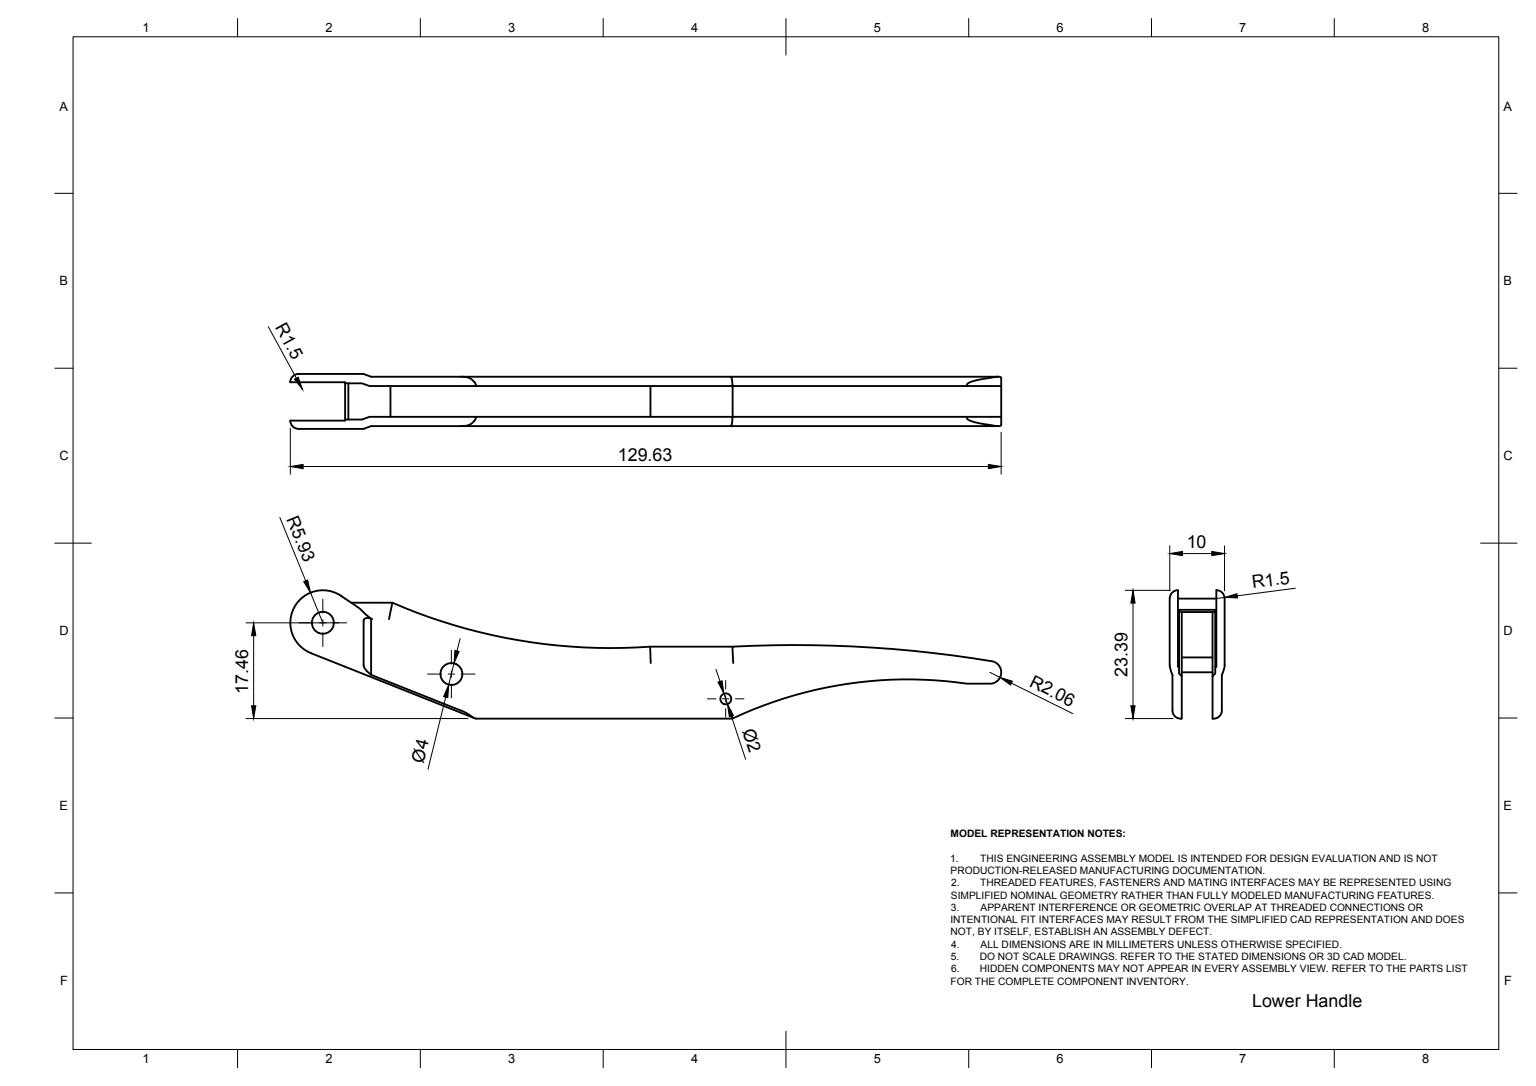
ISO-10303-21;
HEADER;
/* Generated by software containing ST-Developer
 * from STEP Tools, Inc. (www.steptools.com) 
 */

FILE_DESCRIPTION(
/* description */ ('STEP AP214'),
/* implementation_level */ '2;1');

FILE_NAME(
/* name */ 'Lower Handle.step',
/* time_stamp */ '2026-10-06T11:11:25-07:00',
/* author */ (''),
/* organization */ (''),
/* preprocessor_version */ 'ST-DEVELOPER v20.2',
/* originating_system */ 'Autodesk Translation Framework v15.15.0.0',
/* authorisation */ '');

FILE_SCHEMA (('AUTOMOTIVE_DESIGN { 1 0 10303 214 3 1 1 }'));
ENDSEC;

DATA;
#10=MECHANICAL_DESIGN_GEOMETRIC_PRESENTATION_REPRESENTATION('',(#705),#47717);
#113=ELLIPSE('',#9746,4.06396121899487,1.49999999996976);
#114=ELLIPSE('',#9760,4.06396121989312,1.50000000014194);
#115=ELLIPSE('',#9762,4.71890632484228,1.50000000000588);
#116=ELLIPSE('',#9763,5.29011801808111,1.49999999999909);
#117=ELLIPSE('',#9769,4.71890632482846,1.5000000000021);
#118=ELLIPSE('',#9770,5.29011801808671,1.49999999999996);
#119=ELLIPSE('',#9772,5.36487494985319,2.99999999998019);
#120=ELLIPSE('',#9773,5.36487494986476,2.99999999998425);
#471=B_SPLINE_CURVE_WITH_KNOTS('',3,(#45251,#45252,#45253,#45254,#45255,
#45256,#45257,#45258,#45259,#45260,#45261,#45262,#45263,#45264),
 .UNSPECIFIED.,.F.,.F.,(4,2,2,2,2,2,4),(-0.478011466323298,-0.477450068616196,
-0.4160793870133,-0.355479826428422,-0.296403852091954,-0.238674806903838,
-0.238656685114328),.UNSPECIFIED.);
#472=B_SPLINE_CURVE_WITH_KNOTS('',3,(#45268,#45269,#45270,#45271,#45272,
#45273,#45274,#45275),.UNSPECIFIED.,.F.,.F.,(4,2,2,4),(-1.28046581538947,
-1.24694324764166,-1.16660067584426,-1.12172029214894),.UNSPECIFIED.);
#473=B_SPLINE_CURVE_WITH_KNOTS('',3,(#45276,#45277,#45278,#45279,#45280,
#45281,#45282,#45283,#45284,#45285,#45286,#45287),.UNSPECIFIED.,.F.,.F.,
(4,2,2,2,2,4),(1.32320401424985,1.33548572406861,1.3557039818829,1.41353490960294,
1.47136583732297,1.75011843198071),.UNSPECIFIED.);
#474=B_SPLINE_CURVE_WITH_KNOTS('',3,(#45293,#45294,#45295,#45296,#45297,
#45298,#45299,#45300,#45301,#45302,#45303,#45304,#45305,#45306),
 .UNSPECIFIED.,.F.,.F.,(4,2,2,2,2,2,4),(-0.238656685112889,-0.181355245214609,
-0.12330633361927,-0.0637887774894114,-0.0319236327969544,-1.27398092075737E-14,
0.000561480190367634),.UNSPECIFIED.);
#475=B_SPLINE_CURVE_WITH_KNOTS('',3,(#45310,#45311,#45312,#45313,#45314,
#45315,#45316,#45317,#45318,#45319,#45320,#45321),.UNSPECIFIED.,.F.,.F.,
(4,2,2,2,2,4),(0.893026008311947,1.17177860296978,1.22960953068981,1.28744045840985,
1.30765871622413,1.3199404260429),.UNSPECIFIED.);
#476=B_SPLINE_CURVE_WITH_KNOTS('',3,(#45322,#45323,#45324,#45325,#45326,
#45327,#45328,#45329,#45330,#45331),.UNSPECIFIED.,.F.,.F.,(4,2,2,2,4),(-0.624724582317791,
-0.602042604282301,-0.537958860857827,-0.489657632758387,-0.482259949143694),
 .UNSPECIFIED.);
#477=B_SPLINE_CURVE_WITH_KNOTS('',3,(#45337,#45338,#45339,#45340,#45341,
#45342,#45343,#45344,#45345,#45346,#45347,#45348,#45349,#45350,#45351,#45352,
#45353,#45354,#45355,#45356,#45357,#45358),.UNSPECIFIED.,.F.,.F.,(4,2,2,
2,1,1,1,1,2,2,2,2,4),(0.,0.250000000000738,0.375000000001107,0.43750000000129,
0.468750000001377,0.484375000001422,0.492187500001443,0.496093750001453,
0.49804687500145,0.500000000001447,0.750000000000721,0.87500000000036,1.),
 .UNSPECIFIED.);
#478=B_SPLINE_CURVE_WITH_KNOTS('',3,(#45361,#45362,#45363,#45364,#45365,
#45366,#45367,#45368,#45369,#45370,#45371,#45372,#45373,#45374,#45375,#45376),
 .UNSPECIFIED.,.F.,.F.,(4,2,2,2,2,2,2,4),(-0.539155078775716,-0.498671728991868,
-0.431839786572352,-0.357600677552978,-0.261503696582492,-0.134722695832283,
0.,0.0010080897643522),.UNSPECIFIED.);
#479=B_SPLINE_CURVE_WITH_KNOTS('',3,(#45382,#45383,#45384,#45385,#45386,
#45387,#45388,#45389,#45390,#45391,#45392,#45393,#45394,#45395,#45396,#45397,
#45398,#45399,#45400,#45401,#45402,#45403),.UNSPECIFIED.,.F.,.F.,(4,2,2,
2,2,1,1,1,1,2,2,2,4),(0.000307299979407227,0.124999999999807,0.249999999999614,
0.374999999999422,0.437499999999325,0.46874999999927,0.484374999999239,
0.492187499999224,0.496093749999213,0.498046874999211,0.499999999999209,
0.749999999999605,1.),.UNSPECIFIED.);
#480=B_SPLINE_CURVE_WITH_KNOTS('',3,(#45406,#45407,#45408,#45409,#45410,
#45411,#45412,#45413,#45414,#45415,#45416,#45417,#45418,#45419,#45420,#45421),
 .UNSPECIFIED.,.F.,.F.,(4,2,2,2,2,2,2,4),(-1.54028535744593,-1.53927726768737,
-1.40455457263243,-1.27777357261349,-1.18167659219378,-1.10743748360041,
-1.04060554156496,-1.00012219201053),.UNSPECIFIED.);
#481=B_SPLINE_CURVE_WITH_KNOTS('',3,(#45655,#45656,#45657,#45658,#45659,
#45660,#45661,#45662,#45663,#45664,#45665,#45666,#45667,#45668,#45669,#45670,
#45671,#45672,#45673,#45674,#45675,#45676,#45677,#45678,#45679,#45680,#45681,
#45682,#45683,#45684,#45685,#45686,#45687,#45688,#45689,#45690,#45691,#45692,
#45693,#45694,#45695,#45696,#45697,#45698,#45699,#45700,#45701,#45702,#45703,
#45704,#45705,#45706,#45707,#45708,#45709,#45710,#45711,#45712,#45713,#45714,
#45715,#45716,#45717,#45718,#45719,#45720,#45721,#45722,#45723,#45724,#45725,
#45726,#45727),.UNSPECIFIED.,.F.,.F.,(4,3,3,3,3,3,3,3,3,3,3,3,3,3,3,3,3,
3,3,3,3,3,3,3,4),(-4.11257062550913E-5,0.000211162300231747,0.00046350988042877,
0.000715878564535794,0.000968550589332387,0.00114123113312901,0.00138545825899057,
0.00162944378491571,0.00173240955282102,0.0019623825795414,0.00219370350738769,
0.00232358797251303,0.00250954819935604,0.00269528994831476,0.00288121303245579,
0.00291476639220505,0.00314628582243956,0.00337751095812055,0.00350594481189706,
0.00370563324181197,0.00390550571072881,0.00409712323158908,0.00432708598005531,
0.00455518200144187,0.00468830165128109),.UNSPECIFIED.);
#482=B_SPLINE_CURVE_WITH_KNOTS('',3,(#45728,#45729,#45730,#45731,#45732,
#45733,#45734,#45735,#45736,#45737,#45738,#45739,#45740,#45741),
 .UNSPECIFIED.,.F.,.F.,(4,2,2,2,2,2,4),(-0.95463956460269,-0.953847234743663,
-0.831921008082044,-0.711276912435687,-0.593231640056803,-0.477522014556901,
-0.476788308545111),.UNSPECIFIED.);
#483=B_SPLINE_CURVE_WITH_KNOTS('',3,(#45743,#45744,#45745,#45746,#45747,
#45748,#45749,#45750),.UNSPECIFIED.,.F.,.F.,(4,2,2,4),(-1.1200552360125,
-1.06565795604777,-0.91947526211342,-0.773292568179073),.UNSPECIFIED.);
#484=B_SPLINE_CURVE_WITH_KNOTS('',3,(#45752,#45753,#45754,#45755,#45756,
#45757,#45758,#45759,#45760,#45761,#45762,#45763,#45764,#45765,#45766,#45767,
#45768,#45769,#45770,#45771,#45772,#45773,#45774,#45775,#45776,#45777,#45778,
#45779,#45780,#45781,#45782,#45783,#45784,#45785,#45786,#45787,#45788,#45789,
#45790,#45791,#45792,#45793,#45794,#45795,#45796,#45797,#45798,#45799,#45800,
#45801,#45802,#45803,#45804,#45805,#45806,#45807,#45808,#45809,#45810,#45811,
#45812,#45813,#45814,#45815,#45816,#45817,#45818,#45819,#45820,#45821,#45822,
#45823,#45824),.UNSPECIFIED.,.F.,.F.,(4,3,3,3,3,3,3,3,3,3,3,3,3,3,3,3,3,
3,3,3,3,3,3,3,4),(0.,0.000225667550044305,0.000453521175865013,0.00058601050704541,
0.000784129836157538,0.000982083285598081,0.00117202101409082,0.00140097570403084,
0.00163057513263886,0.00175803152113623,0.00194229610832416,0.00212641016209573,
0.00231079586156332,0.00234404202818164,0.00257328610067309,0.00280154068634866,
0.00293005253522705,0.00317214395432889,0.00341450191345266,0.00351606304227246,
0.00384363571960531,0.00410207354931787,0.00429883028119473,0.00449594514523909,
0.00468808405636328),.UNSPECIFIED.);
#485=B_SPLINE_CURVE_WITH_KNOTS('',3,(#45825,#45826,#45827,#45828,#45829,
#45830,#45831,#45832,#45833,#45834,#45835,#45836,#45837,#45838),
 .UNSPECIFIED.,.F.,.F.,(4,2,2,2,2,2,4),(-0.477116828714656,-0.476383034932386,
-0.360659365287303,-0.242599765287782,-0.121941026584239,-2.22044604925031E-15,
0.000792426037240202),.UNSPECIFIED.);
#486=B_SPLINE_CURVE_WITH_KNOTS('',3,(#45840,#45841,#45842,#45843,#45844,
#45845,#45846,#45847),.UNSPECIFIED.,.F.,.F.,(4,2,2,4),(-2.26503183854715,
-2.1188491446128,-1.97266645067846,-1.91826917071372),.UNSPECIFIED.);
#487=B_SPLINE_CURVE_WITH_KNOTS('',3,(#45855,#45856,#45857,#45858,#45859,
#45860,#45861,#45862,#45863,#45864),.UNSPECIFIED.,.F.,.F.,(4,2,2,2,4),(-1.32111970138292,
-1.30631571776553,-1.23358981994045,-1.16086392211537,-1.01541212646521),
 .UNSPECIFIED.);
#488=B_SPLINE_CURVE_WITH_KNOTS('',3,(#45876,#45877,#45878,#45879,#45880,
#45881,#45882,#45883,#45884,#45885),.UNSPECIFIED.,.F.,.F.,(4,2,2,2,4),(-2.36315569877945,
-2.21770390312929,-2.14497800530421,-2.07225210747913,-2.05744812386174),
 .UNSPECIFIED.);
#652=TOROIDAL_SURFACE('',#9704,76.5,1.5);
#653=TOROIDAL_SURFACE('',#9707,76.5,1.5);
#654=TOROIDAL_SURFACE('',#9710,219.,3.);
#655=TOROIDAL_SURFACE('',#9713,219.,3.);
#656=TOROIDAL_SURFACE('',#9788,103.,3.);
#657=TOROIDAL_SURFACE('',#9790,103.,3.);
#658=TOROIDAL_SURFACE('',#9797,4.43478616545488,1.5);
#659=TOROIDAL_SURFACE('',#9804,4.43478616545488,1.5);
#681=SHAPE_REPRESENTATION_RELATIONSHIP('SRR','None',#47768,#693);
#693=ADVANCED_BREP_SHAPE_REPRESENTATION('',(#717),#47712);
#705=STYLED_ITEM('',(#47830),#717);
#717=MANIFOLD_SOLID_BREP('Body1',#8932);
#737=FACE_BOUND('',#2996,.T.);
#738=FACE_BOUND('',#2997,.T.);
#739=FACE_BOUND('',#2999,.T.);
#740=FACE_BOUND('',#3000,.T.);
#741=FACE_BOUND('',#3008,.T.);
#742=FACE_BOUND('',#3010,.T.);
#743=FACE_BOUND('',#3014,.T.);
#744=FACE_BOUND('',#3015,.T.);
#745=FACE_BOUND('',#3017,.T.);
#746=FACE_BOUND('',#3018,.T.);
#747=FACE_BOUND('',#3044,.T.);
#748=FACE_BOUND('',#3046,.T.);
#842=PLANE('',#9742);
#843=PLANE('',#9743);
#844=PLANE('',#9744);
#845=PLANE('',#9745);
#846=PLANE('',#9747);
#847=PLANE('',#9750);
#848=PLANE('',#9753);
#849=PLANE('',#9757);
#850=PLANE('',#9758);
#851=PLANE('',#9759);
#852=PLANE('',#9761);
#853=PLANE('',#9764);
#854=PLANE('',#9766);
#855=PLANE('',#9768);
#856=PLANE('',#9771);
#857=PLANE('',#9774);
#858=PLANE('',#9777);
#859=PLANE('',#9780);
#860=PLANE('',#9782);
#861=PLANE('',#9783);
#862=PLANE('',#9784);
#863=PLANE('',#9785);
#864=PLANE('',#9786);
#865=PLANE('',#9787);
#866=PLANE('',#9809);
#867=PLANE('',#9810);
#868=PLANE('',#9811);
#1241=LINE('',#45427,#1728);
#1242=LINE('',#45430,#1729);
#1243=LINE('',#45435,#1730);
#1244=LINE('',#45441,#1731);
#1245=LINE('',#45447,#1732);
#1246=LINE('',#45451,#1733);
#1247=LINE('',#45454,#1734);
#1248=LINE('',#45459,#1735);
#1249=LINE('',#45465,#1736);
#1250=LINE('',#45471,#1737);
#1251=LINE('',#45477,#1738);
#1252=LINE('',#45478,#1739);
#1253=LINE('',#45480,#1740);
#1254=LINE('',#45481,#1741);
#1255=LINE('',#45484,#1742);
#1256=LINE('',#45485,#1743);
#1257=LINE('',#45488,#1744);
#1258=LINE('',#45489,#1745);
#1259=LINE('',#45492,#1746);
#1260=LINE('',#45494,#1747);
#1261=LINE('',#45495,#1748);
#1262=LINE('',#45499,#1749);
#1263=LINE('',#45501,#1750);
#1264=LINE('',#45503,#1751);
#1265=LINE('',#45505,#1752);
#1266=LINE('',#45506,#1753);
#1267=LINE('',#45511,#1754);
#1268=LINE('',#45513,#1755);
#1269=LINE('',#45515,#1756);
#1270=LINE('',#45517,#1757);
#1271=LINE('',#45519,#1758);
#1272=LINE('',#45522,#1759);
#1273=LINE('',#45526,#1760);
#1274=LINE('',#45530,#1761);
#1275=LINE('',#45532,#1762);
#1276=LINE('',#45534,#1763);
#1277=LINE('',#45536,#1764);
#1278=LINE('',#45537,#1765);
#1279=LINE('',#45541,#1766);
#1280=LINE('',#45543,#1767);
#1281=LINE('',#45545,#1768);
#1282=LINE('',#45546,#1769);
#1283=LINE('',#45551,#1770);
#1284=LINE('',#45554,#1771);
#1285=LINE('',#45555,#1772);
#1286=LINE('',#45559,#1773);
#1287=LINE('',#45560,#1774);
#1288=LINE('',#45561,#1775);
#1289=LINE('',#45565,#1776);
#1290=LINE('',#45567,#1777);
#1291=LINE('',#45569,#1778);
#1292=LINE('',#45572,#1779);
#1293=LINE('',#45573,#1780);
#1294=LINE('',#45577,#1781);
#1295=LINE('',#45583,#1782);
#1296=LINE('',#45585,#1783);
#1297=LINE('',#45588,#1784);
#1298=LINE('',#45593,#1785);
#1299=LINE('',#45594,#1786);
#1300=LINE('',#45601,#1787);
#1301=LINE('',#45603,#1788);
#1302=LINE('',#45605,#1789);
#1303=LINE('',#45611,#1790);
#1304=LINE('',#45615,#1791);
#1305=LINE('',#45616,#1792);
#1306=LINE('',#45620,#1793);
#1307=LINE('',#45622,#1794);
#1308=LINE('',#45625,#1795);
#1309=LINE('',#45628,#1796);
#1310=LINE('',#45630,#1797);
#1311=LINE('',#45632,#1798);
#1312=LINE('',#45634,#1799);
#1313=LINE('',#45635,#1800);
#1314=LINE('',#45636,#1801);
#1315=LINE('',#45638,#1802);
#1316=LINE('',#45641,#1803);
#1317=LINE('',#45644,#1804);
#1318=LINE('',#45645,#1805);
#1319=LINE('',#45646,#1806);
#1320=LINE('',#45649,#1807);
#1321=LINE('',#45650,#1808);
#1322=LINE('',#45653,#1809);
#1323=LINE('',#45852,#1810);
#1324=LINE('',#45870,#1811);
#1325=LINE('',#45874,#1812);
#1326=LINE('',#45891,#1813);
#1327=LINE('',#45894,#1814);
#1328=LINE('',#45895,#1815);
#1728=VECTOR('',#11610,1000.);
#1729=VECTOR('',#11613,1000.);
#1730=VECTOR('',#11618,2.);
#1731=VECTOR('',#11625,2.);
#1732=VECTOR('',#11632,1.00000000000001);
#1733=VECTOR('',#11637,1000.);
#1734=VECTOR('',#11640,1000.);
#1735=VECTOR('',#11645,2.);
#1736=VECTOR('',#11652,2.);
#1737=VECTOR('',#11659,1.00000000000001);
#1738=VECTOR('',#11666,1000.);
#1739=VECTOR('',#11667,1000.);
#1740=VECTOR('',#11670,1000.);
#1741=VECTOR('',#11671,1000.);
#1742=VECTOR('',#11674,1000.);
#1743=VECTOR('',#11675,1000.);
#1744=VECTOR('',#11678,1000.);
#1745=VECTOR('',#11679,1000.);
#1746=VECTOR('',#11682,1000.);
#1747=VECTOR('',#11683,1000.);
#1748=VECTOR('',#11684,1000.);
#1749=VECTOR('',#11687,1000.);
#1750=VECTOR('',#11688,1000.);
#1751=VECTOR('',#11689,1000.);
#1752=VECTOR('',#11690,1000.);
#1753=VECTOR('',#11691,1000.);
#1754=VECTOR('',#11698,1000.);
#1755=VECTOR('',#11699,1000.);
#1756=VECTOR('',#11700,1000.);
#1757=VECTOR('',#11701,1000.);
#1758=VECTOR('',#11702,1000.);
#1759=VECTOR('',#11705,1000.);
#1760=VECTOR('',#11710,1000.);
#1761=VECTOR('',#11713,1000.);
#1762=VECTOR('',#11714,1000.);
#1763=VECTOR('',#11715,1000.);
#1764=VECTOR('',#11716,1000.);
#1765=VECTOR('',#11717,1000.);
#1766=VECTOR('',#11720,1000.);
#1767=VECTOR('',#11721,1000.);
#1768=VECTOR('',#11722,1000.);
#1769=VECTOR('',#11723,1000.);
#1770=VECTOR('',#11728,1000.);
#1771=VECTOR('',#11733,1000.);
#1772=VECTOR('',#11734,1000.);
#1773=VECTOR('',#11737,1000.);
#1774=VECTOR('',#11738,1000.);
#1775=VECTOR('',#11739,1000.);
#1776=VECTOR('',#11742,1000.);
#1777=VECTOR('',#11743,1000.);
#1778=VECTOR('',#11744,1000.);
#1779=VECTOR('',#11747,1000.);
#1780=VECTOR('',#11748,1000.);
#1781=VECTOR('',#11751,1000.);
#1782=VECTOR('',#11758,1000.);
#1783=VECTOR('',#11759,1000.);
#1784=VECTOR('',#11762,1000.);
#1785=VECTOR('',#11767,1000.);
#1786=VECTOR('',#11768,1000.);
#1787=VECTOR('',#11777,1000.);
#1788=VECTOR('',#11778,1000.);
#1789=VECTOR('',#11779,1000.);
#1790=VECTOR('',#11788,1000.);
#1791=VECTOR('',#11791,1000.);
#1792=VECTOR('',#11792,1000.);
#1793=VECTOR('',#11797,1000.);
#1794=VECTOR('',#11798,1000.);
#1795=VECTOR('',#11801,1000.);
#1796=VECTOR('',#11804,1000.);
#1797=VECTOR('',#11805,1000.);
#1798=VECTOR('',#11806,1000.);
#1799=VECTOR('',#11807,1000.);
#1800=VECTOR('',#11808,1000.);
#1801=VECTOR('',#11809,1000.);
#1802=VECTOR('',#11812,1000.);
#1803=VECTOR('',#11817,1000.);
#1804=VECTOR('',#11820,1000.);
#1805=VECTOR('',#11821,1000.);
#1806=VECTOR('',#11822,1000.);
#1807=VECTOR('',#11825,1000.);
#1808=VECTOR('',#11826,1000.);
#1809=VECTOR('',#11831,1000.);
#1810=VECTOR('',#11846,1000.);
#1811=VECTOR('',#11859,1000.);
#1812=VECTOR('',#11864,1000.);
#1813=VECTOR('',#11875,1000.);
#1814=VECTOR('',#11880,1000.);
#1815=VECTOR('',#11881,1000.);
#2017=CYLINDRICAL_SURFACE('',#9716,220.3);
#2018=CYLINDRICAL_SURFACE('',#9719,2.);
#2019=CYLINDRICAL_SURFACE('',#9722,2.);
#2020=CYLINDRICAL_SURFACE('',#9725,1.00000000000001);
#2021=CYLINDRICAL_SURFACE('',#9728,75.);
#2022=CYLINDRICAL_SURFACE('',#9730,2.);
#2023=CYLINDRICAL_SURFACE('',#9733,2.);
#2024=CYLINDRICAL_SURFACE('',#9736,1.00000000000001);
#2025=CYLINDRICAL_SURFACE('',#9739,75.);
#2026=CYLINDRICAL_SURFACE('',#9741,222.);
#2027=CYLINDRICAL_SURFACE('',#9754,100.);
#2028=CYLINDRICAL_SURFACE('',#9781,101.7);
#2029=CYLINDRICAL_SURFACE('',#9789,3.);
#2030=CYLINDRICAL_SURFACE('',#9791,3.00000000000001);
#2031=CYLINDRICAL_SURFACE('',#9792,3.00000000000001);
#2032=CYLINDRICAL_SURFACE('',#9793,3.00000000000001);
#2033=CYLINDRICAL_SURFACE('',#9794,1.5);
#2034=CYLINDRICAL_SURFACE('',#9796,1.5);
#2035=CYLINDRICAL_SURFACE('',#9800,1.5);
#2036=CYLINDRICAL_SURFACE('',#9801,1.5);
#2037=CYLINDRICAL_SURFACE('',#9803,1.5);
#2038=CYLINDRICAL_SURFACE('',#9807,1.5);
#2039=CYLINDRICAL_SURFACE('',#9808,2.06253449527014);
#2450=FACE_OUTER_BOUND('',#2977,.T.);
#2451=FACE_OUTER_BOUND('',#2978,.T.);
#2452=FACE_OUTER_BOUND('',#2979,.T.);
#2453=FACE_OUTER_BOUND('',#2980,.T.);
#2454=FACE_OUTER_BOUND('',#2981,.T.);
#2455=FACE_OUTER_BOUND('',#2982,.T.);
#2456=FACE_OUTER_BOUND('',#2983,.T.);
#2457=FACE_OUTER_BOUND('',#2984,.T.);
#2458=FACE_OUTER_BOUND('',#2985,.T.);
#2459=FACE_OUTER_BOUND('',#2986,.T.);
#2460=FACE_OUTER_BOUND('',#2987,.T.);
#2461=FACE_OUTER_BOUND('',#2988,.T.);
#2462=FACE_OUTER_BOUND('',#2989,.T.);
#2463=FACE_OUTER_BOUND('',#2990,.T.);
#2464=FACE_OUTER_BOUND('',#2991,.T.);
#2465=FACE_OUTER_BOUND('',#2992,.T.);
#2466=FACE_OUTER_BOUND('',#2993,.T.);
#2467=FACE_OUTER_BOUND('',#2994,.T.);
#2468=FACE_OUTER_BOUND('',#2995,.T.);
#2469=FACE_OUTER_BOUND('',#2998,.T.);
#2470=FACE_OUTER_BOUND('',#3001,.T.);
#2471=FACE_OUTER_BOUND('',#3002,.T.);
#2472=FACE_OUTER_BOUND('',#3003,.T.);
#2473=FACE_OUTER_BOUND('',#3004,.T.);
#2474=FACE_OUTER_BOUND('',#3005,.T.);
#2475=FACE_OUTER_BOUND('',#3006,.T.);
#2476=FACE_OUTER_BOUND('',#3007,.T.);
#2477=FACE_OUTER_BOUND('',#3009,.T.);
#2478=FACE_OUTER_BOUND('',#3011,.T.);
#2479=FACE_OUTER_BOUND('',#3012,.T.);
#2480=FACE_OUTER_BOUND('',#3013,.T.);
#2481=FACE_OUTER_BOUND('',#3016,.T.);
#2482=FACE_OUTER_BOUND('',#3019,.T.);
#2483=FACE_OUTER_BOUND('',#3020,.T.);
#2484=FACE_OUTER_BOUND('',#3021,.T.);
#2485=FACE_OUTER_BOUND('',#3022,.T.);
#2486=FACE_OUTER_BOUND('',#3023,.T.);
#2487=FACE_OUTER_BOUND('',#3024,.T.);
#2488=FACE_OUTER_BOUND('',#3025,.T.);
#2489=FACE_OUTER_BOUND('',#3026,.T.);
#2490=FACE_OUTER_BOUND('',#3027,.T.);
#2491=FACE_OUTER_BOUND('',#3028,.T.);
#2492=FACE_OUTER_BOUND('',#3029,.T.);
#2493=FACE_OUTER_BOUND('',#3030,.T.);
#2494=FACE_OUTER_BOUND('',#3031,.T.);
#2495=FACE_OUTER_BOUND('',#3032,.T.);
#2496=FACE_OUTER_BOUND('',#3033,.T.);
#2497=FACE_OUTER_BOUND('',#3034,.T.);
#2498=FACE_OUTER_BOUND('',#3035,.T.);
#2499=FACE_OUTER_BOUND('',#3036,.T.);
#2500=FACE_OUTER_BOUND('',#3037,.T.);
#2501=FACE_OUTER_BOUND('',#3038,.T.);
#2502=FACE_OUTER_BOUND('',#3039,.T.);
#2503=FACE_OUTER_BOUND('',#3040,.T.);
#2504=FACE_OUTER_BOUND('',#3041,.T.);
#2505=FACE_OUTER_BOUND('',#3042,.T.);
#2506=FACE_OUTER_BOUND('',#3043,.T.);
#2507=FACE_OUTER_BOUND('',#3045,.T.);
#2977=EDGE_LOOP('',(#7789,#7790,#7791,#7792,#7793));
#2978=EDGE_LOOP('',(#7794,#7795,#7796,#7797,#7798));
#2979=EDGE_LOOP('',(#7799,#7800,#7801,#7802));
#2980=EDGE_LOOP('',(#7803,#7804,#7805,#7806));
#2981=EDGE_LOOP('',(#7807,#7808,#7809,#7810));
#2982=EDGE_LOOP('',(#7811,#7812,#7813,#7814));
#2983=EDGE_LOOP('',(#7815,#7816,#7817,#7818));
#2984=EDGE_LOOP('',(#7819,#7820,#7821,#7822));
#2985=EDGE_LOOP('',(#7823,#7824,#7825,#7826));
#2986=EDGE_LOOP('',(#7827,#7828,#7829,#7830));
#2987=EDGE_LOOP('',(#7831,#7832,#7833,#7834));
#2988=EDGE_LOOP('',(#7835,#7836,#7837,#7838));
#2989=EDGE_LOOP('',(#7839,#7840,#7841,#7842));
#2990=EDGE_LOOP('',(#7843,#7844,#7845,#7846));
#2991=EDGE_LOOP('',(#7847,#7848,#7849,#7850));
#2992=EDGE_LOOP('',(#7851,#7852,#7853,#7854));
#2993=EDGE_LOOP('',(#7855,#7856,#7857,#7858));
#2994=EDGE_LOOP('',(#7859,#7860,#7861,#7862,#7863,#7864,#7865));
#2995=EDGE_LOOP('',(#7866,#7867,#7868,#7869,#7870,#7871,#7872,#7873,#7874,
#7875));
#2996=EDGE_LOOP('',(#7876));
#2997=EDGE_LOOP('',(#7877));
#2998=EDGE_LOOP('',(#7878,#7879,#7880,#7881,#7882,#7883,#7884,#7885,#7886,
#7887));
#2999=EDGE_LOOP('',(#7888));
#3000=EDGE_LOOP('',(#7889));
#3001=EDGE_LOOP('',(#7890,#7891,#7892,#7893));
#3002=EDGE_LOOP('',(#7894,#7895,#7896,#7897));
#3003=EDGE_LOOP('',(#7898,#7899,#7900,#7901));
#3004=EDGE_LOOP('',(#7902,#7903,#7904,#7905));
#3005=EDGE_LOOP('',(#7906,#7907,#7908,#7909,#7910,#7911,#7912));
#3006=EDGE_LOOP('',(#7913,#7914,#7915,#7916));
#3007=EDGE_LOOP('',(#7917,#7918,#7919,#7920));
#3008=EDGE_LOOP('',(#7921));
#3009=EDGE_LOOP('',(#7922,#7923,#7924,#7925));
#3010=EDGE_LOOP('',(#7926));
#3011=EDGE_LOOP('',(#7927,#7928,#7929,#7930));
#3012=EDGE_LOOP('',(#7931,#7932,#7933,#7934,#7935,#7936));
#3013=EDGE_LOOP('',(#7937,#7938,#7939,#7940,#7941,#7942,#7943,#7944,#7945,
#7946));
#3014=EDGE_LOOP('',(#7947));
#3015=EDGE_LOOP('',(#7948));
#3016=EDGE_LOOP('',(#7949,#7950,#7951,#7952,#7953,#7954,#7955,#7956,#7957,
#7958));
#3017=EDGE_LOOP('',(#7959));
#3018=EDGE_LOOP('',(#7960));
#3019=EDGE_LOOP('',(#7961,#7962,#7963,#7964,#7965,#7966,#7967,#7968));
#3020=EDGE_LOOP('',(#7969,#7970,#7971,#7972));
#3021=EDGE_LOOP('',(#7973,#7974,#7975,#7976));
#3022=EDGE_LOOP('',(#7977,#7978,#7979,#7980));
#3023=EDGE_LOOP('',(#7981,#7982,#7983,#7984,#7985));
#3024=EDGE_LOOP('',(#7986,#7987,#7988,#7989,#7990));
#3025=EDGE_LOOP('',(#7991,#7992,#7993,#7994));
#3026=EDGE_LOOP('',(#7995,#7996,#7997,#7998));
#3027=EDGE_LOOP('',(#7999,#8000,#8001,#8002));
#3028=EDGE_LOOP('',(#8003,#8004,#8005,#8006,#8007));
#3029=EDGE_LOOP('',(#8008,#8009,#8010,#8011));
#3030=EDGE_LOOP('',(#8012,#8013,#8014,#8015,#8016));
#3031=EDGE_LOOP('',(#8017,#8018,#8019,#8020));
#3032=EDGE_LOOP('',(#8021,#8022,#8023,#8024));
#3033=EDGE_LOOP('',(#8025,#8026,#8027,#8028,#8029,#8030,#8031));
#3034=EDGE_LOOP('',(#8032,#8033,#8034,#8035,#8036));
#3035=EDGE_LOOP('',(#8037,#8038,#8039,#8040));
#3036=EDGE_LOOP('',(#8041,#8042,#8043,#8044,#8045,#8046,#8047));
#3037=EDGE_LOOP('',(#8048,#8049,#8050,#8051,#8052,#8053,#8054));
#3038=EDGE_LOOP('',(#8055,#8056,#8057,#8058,#8059));
#3039=EDGE_LOOP('',(#8060,#8061,#8062,#8063));
#3040=EDGE_LOOP('',(#8064,#8065,#8066,#8067,#8068,#8069,#8070));
#3041=EDGE_LOOP('',(#8071,#8072,#8073,#8074,#8075,#8076,#8077,#8078,#8079,
#8080,#8081,#8082));
#3042=EDGE_LOOP('',(#8083,#8084,#8085,#8086,#8087,#8088,#8089,#8090));
#3043=EDGE_LOOP('',(#8091,#8092,#8093,#8094));
#3044=EDGE_LOOP('',(#8095));
#3045=EDGE_LOOP('',(#8096,#8097,#8098,#8099));
#3046=EDGE_LOOP('',(#8100));
#3420=CIRCLE('',#9705,75.);
#3421=CIRCLE('',#9706,76.5);
#3422=CIRCLE('',#9708,76.5);
#3423=CIRCLE('',#9709,75.);
#3424=CIRCLE('',#9711,219.);
#3425=CIRCLE('',#9712,222.);
#3426=CIRCLE('',#9714,222.);
#3427=CIRCLE('',#9715,219.);
#3428=CIRCLE('',#9717,220.3);
#3429=CIRCLE('',#9718,220.3);
#3430=CIRCLE('',#9720,2.);
#3431=CIRCLE('',#9721,2.);
#3432=CIRCLE('',#9723,2.);
#3433=CIRCLE('',#9724,2.);
#3434=CIRCLE('',#9726,1.00000000000001);
#3435=CIRCLE('',#9727,1.00000000000001);
#3436=CIRCLE('',#9729,75.);
#3437=CIRCLE('',#9731,2.);
#3438=CIRCLE('',#9732,2.);
#3439=CIRCLE('',#9734,2.);
#3440=CIRCLE('',#9735,2.);
#3441=CIRCLE('',#9737,1.00000000000001);
#3442=CIRCLE('',#9738,1.00000000000001);
#3443=CIRCLE('',#9740,75.);
#3444=CIRCLE('',#9748,2.06253449527014);
#3445=CIRCLE('',#9749,103.);
#3446=CIRCLE('',#9751,2.06253449527014);
#3447=CIRCLE('',#9752,103.);
#3448=CIRCLE('',#9755,100.);
#3449=CIRCLE('',#9756,100.);
#3450=CIRCLE('',#9765,4.43478616545489);
#3451=CIRCLE('',#9767,4.43478616545489);
#3452=CIRCLE('',#9775,2.06253449527014);
#3453=CIRCLE('',#9776,101.7);
#3454=CIRCLE('',#9778,2.06253449527014);
#3455=CIRCLE('',#9779,101.7);
#3456=CIRCLE('',#9795,1.5);
#3457=CIRCLE('',#9798,5.93478616545488);
#3458=CIRCLE('',#9799,1.5);
#3459=CIRCLE('',#9802,1.5);
#3460=CIRCLE('',#9805,1.5);
#3461=CIRCLE('',#9806,5.93478616545488);
#4195=VERTEX_POINT('',#45247);
#4196=VERTEX_POINT('',#45248);
#4197=VERTEX_POINT('',#45250);
#4198=VERTEX_POINT('',#45265);
#4199=VERTEX_POINT('',#45267);
#4200=VERTEX_POINT('',#45289);
#4201=VERTEX_POINT('',#45290);
#4202=VERTEX_POINT('',#45292);
#4203=VERTEX_POINT('',#45307);
#4204=VERTEX_POINT('',#45309);
#4205=VERTEX_POINT('',#45333);
#4206=VERTEX_POINT('',#45334);
#4207=VERTEX_POINT('',#45336);
#4208=VERTEX_POINT('',#45359);
#4209=VERTEX_POINT('',#45378);
#4210=VERTEX_POINT('',#45379);
#4211=VERTEX_POINT('',#45381);
#4212=VERTEX_POINT('',#45404);
#4213=VERTEX_POINT('',#45423);
#4214=VERTEX_POINT('',#45424);
#4215=VERTEX_POINT('',#45426);
#4216=VERTEX_POINT('',#45428);
#4217=VERTEX_POINT('',#45432);
#4218=VERTEX_POINT('',#45434);
#4219=VERTEX_POINT('',#45438);
#4220=VERTEX_POINT('',#45440);
#4221=VERTEX_POINT('',#45444);
#4222=VERTEX_POINT('',#45446);
#4223=VERTEX_POINT('',#45450);
#4224=VERTEX_POINT('',#45452);
#4225=VERTEX_POINT('',#45456);
#4226=VERTEX_POINT('',#45458);
#4227=VERTEX_POINT('',#45462);
#4228=VERTEX_POINT('',#45464);
#4229=VERTEX_POINT('',#45468);
#4230=VERTEX_POINT('',#45470);
#4231=VERTEX_POINT('',#45474);
#4232=VERTEX_POINT('',#45475);
#4233=VERTEX_POINT('',#45483);
#4234=VERTEX_POINT('',#45487);
#4235=VERTEX_POINT('',#45491);
#4236=VERTEX_POINT('',#45493);
#4237=VERTEX_POINT('',#45497);
#4238=VERTEX_POINT('',#45498);
#4239=VERTEX_POINT('',#45500);
#4240=VERTEX_POINT('',#45502);
#4241=VERTEX_POINT('',#45504);
#4242=VERTEX_POINT('',#45510);
#4243=VERTEX_POINT('',#45512);
#4244=VERTEX_POINT('',#45514);
#4245=VERTEX_POINT('',#45516);
#4246=VERTEX_POINT('',#45518);
#4247=VERTEX_POINT('',#45520);
#4248=VERTEX_POINT('',#45525);
#4249=VERTEX_POINT('',#45527);
#4250=VERTEX_POINT('',#45529);
#4251=VERTEX_POINT('',#45531);
#4252=VERTEX_POINT('',#45533);
#4253=VERTEX_POINT('',#45535);
#4254=VERTEX_POINT('',#45539);
#4255=VERTEX_POINT('',#45540);
#4256=VERTEX_POINT('',#45542);
#4257=VERTEX_POINT('',#45544);
#4258=VERTEX_POINT('',#45548);
#4259=VERTEX_POINT('',#45550);
#4260=VERTEX_POINT('',#45557);
#4261=VERTEX_POINT('',#45558);
#4262=VERTEX_POINT('',#45563);
#4263=VERTEX_POINT('',#45564);
#4264=VERTEX_POINT('',#45566);
#4265=VERTEX_POINT('',#45568);
#4266=VERTEX_POINT('',#45571);
#4267=VERTEX_POINT('',#45575);
#4268=VERTEX_POINT('',#45576);
#4269=VERTEX_POINT('',#45581);
#4270=VERTEX_POINT('',#45582);
#4271=VERTEX_POINT('',#45584);
#4272=VERTEX_POINT('',#45586);
#4273=VERTEX_POINT('',#45590);
#4274=VERTEX_POINT('',#45591);
#4275=VERTEX_POINT('',#45599);
#4276=VERTEX_POINT('',#45600);
#4277=VERTEX_POINT('',#45602);
#4278=VERTEX_POINT('',#45604);
#4279=VERTEX_POINT('',#45610);
#4280=VERTEX_POINT('',#45612);
#4281=VERTEX_POINT('',#45614);
#4282=VERTEX_POINT('',#45619);
#4283=VERTEX_POINT('',#45621);
#4284=VERTEX_POINT('',#45623);
#4285=VERTEX_POINT('',#45627);
#4286=VERTEX_POINT('',#45629);
#4287=VERTEX_POINT('',#45631);
#4288=VERTEX_POINT('',#45633);
#4289=VERTEX_POINT('',#45643);
#4290=VERTEX_POINT('',#45648);
#4291=VERTEX_POINT('',#45851);
#4292=VERTEX_POINT('',#45866);
#4293=VERTEX_POINT('',#45872);
#4294=VERTEX_POINT('',#45887);
#5420=EDGE_CURVE('',#4195,#4196,#3420,.T.);
#5421=EDGE_CURVE('',#4197,#4195,#471,.T.);
#5422=EDGE_CURVE('',#4198,#4197,#3421,.T.);
#5423=EDGE_CURVE('',#4199,#4198,#472,.T.);
#5424=EDGE_CURVE('',#4196,#4199,#473,.T.);
#5425=EDGE_CURVE('',#4200,#4201,#3422,.T.);
#5426=EDGE_CURVE('',#4202,#4200,#474,.T.);
#5427=EDGE_CURVE('',#4203,#4202,#3423,.T.);
#5428=EDGE_CURVE('',#4204,#4203,#475,.T.);
#5429=EDGE_CURVE('',#4201,#4204,#476,.T.);
#5430=EDGE_CURVE('',#4205,#4206,#3424,.T.);
#5431=EDGE_CURVE('',#4207,#4205,#477,.T.);
#5432=EDGE_CURVE('',#4208,#4207,#3425,.T.);
#5433=EDGE_CURVE('',#4206,#4208,#478,.T.);
#5434=EDGE_CURVE('',#4209,#4210,#3426,.T.);
#5435=EDGE_CURVE('',#4211,#4209,#479,.T.);
#5436=EDGE_CURVE('',#4212,#4211,#3427,.T.);
#5437=EDGE_CURVE('',#4210,#4212,#480,.T.);
#5438=EDGE_CURVE('',#4213,#4214,#3428,.T.);
#5439=EDGE_CURVE('',#4215,#4214,#1241,.T.);
#5440=EDGE_CURVE('',#4216,#4215,#3429,.T.);
#5441=EDGE_CURVE('',#4213,#4216,#1242,.T.);
#5442=EDGE_CURVE('',#4217,#4217,#3430,.T.);
#5443=EDGE_CURVE('',#4217,#4218,#1243,.T.);
#5444=EDGE_CURVE('',#4218,#4218,#3431,.T.);
#5445=EDGE_CURVE('',#4219,#4219,#3432,.T.);
#5446=EDGE_CURVE('',#4219,#4220,#1244,.T.);
#5447=EDGE_CURVE('',#4220,#4220,#3433,.T.);
#5448=EDGE_CURVE('',#4221,#4221,#3434,.T.);
#5449=EDGE_CURVE('',#4221,#4222,#1245,.T.);
#5450=EDGE_CURVE('',#4222,#4222,#3435,.T.);
#5451=EDGE_CURVE('',#4196,#4223,#1246,.T.);
#5452=EDGE_CURVE('',#4223,#4224,#3436,.T.);
#5453=EDGE_CURVE('',#4195,#4224,#1247,.T.);
#5454=EDGE_CURVE('',#4225,#4225,#3437,.T.);
#5455=EDGE_CURVE('',#4225,#4226,#1248,.T.);
#5456=EDGE_CURVE('',#4226,#4226,#3438,.T.);
#5457=EDGE_CURVE('',#4227,#4227,#3439,.T.);
#5458=EDGE_CURVE('',#4227,#4228,#1249,.T.);
#5459=EDGE_CURVE('',#4228,#4228,#3440,.T.);
#5460=EDGE_CURVE('',#4229,#4229,#3441,.T.);
#5461=EDGE_CURVE('',#4229,#4230,#1250,.T.);
#5462=EDGE_CURVE('',#4230,#4230,#3442,.T.);
#5463=EDGE_CURVE('',#4231,#4232,#3443,.T.);
#5464=EDGE_CURVE('',#4231,#4203,#1251,.T.);
#5465=EDGE_CURVE('',#4232,#4202,#1252,.T.);
#5466=EDGE_CURVE('',#4207,#4209,#1253,.T.);
#5467=EDGE_CURVE('',#4208,#4210,#1254,.T.);
#5468=EDGE_CURVE('',#4233,#4204,#1255,.T.);
#5469=EDGE_CURVE('',#4233,#4231,#1256,.T.);
#5470=EDGE_CURVE('',#4199,#4234,#1257,.T.);
#5471=EDGE_CURVE('',#4234,#4223,#1258,.T.);
#5472=EDGE_CURVE('',#4202,#4235,#1259,.T.);
#5473=EDGE_CURVE('',#4236,#4235,#1260,.T.);
#5474=EDGE_CURVE('',#4232,#4236,#1261,.T.);
#5475=EDGE_CURVE('',#4237,#4238,#1262,.T.);
#5476=EDGE_CURVE('',#4238,#4239,#1263,.T.);
#5477=EDGE_CURVE('',#4240,#4239,#1264,.T.);
#5478=EDGE_CURVE('',#4241,#4240,#1265,.T.);
#5479=EDGE_CURVE('',#4236,#4241,#1266,.T.);
#5480=EDGE_CURVE('',#4235,#4237,#113,.T.);
#5481=EDGE_CURVE('',#4206,#4198,#3444,.T.);
#5482=EDGE_CURVE('',#4197,#4242,#1267,.T.);
#5483=EDGE_CURVE('',#4242,#4243,#1268,.T.);
#5484=EDGE_CURVE('',#4243,#4244,#1269,.T.);
#5485=EDGE_CURVE('',#4244,#4245,#1270,.T.);
#5486=EDGE_CURVE('',#4245,#4246,#1271,.T.);
#5487=EDGE_CURVE('',#4246,#4247,#3445,.T.);
#5488=EDGE_CURVE('',#4247,#4205,#1272,.T.);
#5489=EDGE_CURVE('',#4212,#4201,#3446,.T.);
#5490=EDGE_CURVE('',#4211,#4248,#1273,.T.);
#5491=EDGE_CURVE('',#4248,#4249,#3447,.T.);
#5492=EDGE_CURVE('',#4249,#4250,#1274,.T.);
#5493=EDGE_CURVE('',#4250,#4251,#1275,.T.);
#5494=EDGE_CURVE('',#4252,#4251,#1276,.T.);
#5495=EDGE_CURVE('',#4252,#4253,#1277,.T.);
#5496=EDGE_CURVE('',#4253,#4200,#1278,.T.);
#5497=EDGE_CURVE('',#4254,#4255,#1279,.T.);
#5498=EDGE_CURVE('',#4255,#4256,#1280,.T.);
#5499=EDGE_CURVE('',#4257,#4256,#1281,.T.);
#5500=EDGE_CURVE('',#4257,#4254,#1282,.T.);
#5501=EDGE_CURVE('',#4256,#4258,#3448,.T.);
#5502=EDGE_CURVE('',#4259,#4258,#1283,.T.);
#5503=EDGE_CURVE('',#4259,#4257,#3449,.T.);
#5504=EDGE_CURVE('',#4258,#4209,#1284,.T.);
#5505=EDGE_CURVE('',#4207,#4259,#1285,.T.);
#5506=EDGE_CURVE('',#4260,#4261,#1286,.T.);
#5507=EDGE_CURVE('',#4260,#4195,#1287,.T.);
#5508=EDGE_CURVE('',#4224,#4261,#1288,.T.);
#5509=EDGE_CURVE('',#4262,#4263,#1289,.T.);
#5510=EDGE_CURVE('',#4263,#4264,#1290,.T.);
#5511=EDGE_CURVE('',#4264,#4265,#1291,.T.);
#5512=EDGE_CURVE('',#4265,#4260,#114,.T.);
#5513=EDGE_CURVE('',#4261,#4266,#1292,.T.);
#5514=EDGE_CURVE('',#4262,#4266,#1293,.T.);
#5515=EDGE_CURVE('',#4267,#4268,#1294,.T.);
#5516=EDGE_CURVE('',#4268,#4252,#115,.T.);
#5517=EDGE_CURVE('',#4251,#4267,#116,.T.);
#5518=EDGE_CURVE('',#4269,#4270,#1295,.T.);
#5519=EDGE_CURVE('',#4270,#4271,#1296,.T.);
#5520=EDGE_CURVE('',#4271,#4272,#3450,.T.);
#5521=EDGE_CURVE('',#4272,#4269,#1297,.T.);
#5522=EDGE_CURVE('',#4273,#4274,#3451,.T.);
#5523=EDGE_CURVE('',#4274,#4268,#1298,.T.);
#5524=EDGE_CURVE('',#4267,#4273,#1299,.T.);
#5525=EDGE_CURVE('',#4243,#4270,#117,.T.);
#5526=EDGE_CURVE('',#4269,#4244,#118,.T.);
#5527=EDGE_CURVE('',#4275,#4276,#1300,.T.);
#5528=EDGE_CURVE('',#4276,#4277,#1301,.T.);
#5529=EDGE_CURVE('',#4277,#4278,#1302,.T.);
#5530=EDGE_CURVE('',#4278,#4255,#119,.T.);
#5531=EDGE_CURVE('',#4254,#4275,#120,.T.);
#5532=EDGE_CURVE('',#4214,#4234,#3452,.T.);
#5533=EDGE_CURVE('',#4279,#4213,#1303,.T.);
#5534=EDGE_CURVE('',#4280,#4279,#3453,.T.);
#5535=EDGE_CURVE('',#4281,#4280,#1304,.T.);
#5536=EDGE_CURVE('',#4266,#4281,#1305,.T.);
#5537=EDGE_CURVE('',#4215,#4233,#3454,.T.);
#5538=EDGE_CURVE('',#4241,#4282,#1306,.T.);
#5539=EDGE_CURVE('',#4282,#4283,#1307,.T.);
#5540=EDGE_CURVE('',#4283,#4284,#3455,.T.);
#5541=EDGE_CURVE('',#4284,#4216,#1308,.T.);
#5542=EDGE_CURVE('',#4282,#4285,#1309,.T.);
#5543=EDGE_CURVE('',#4286,#4285,#1310,.T.);
#5544=EDGE_CURVE('',#4287,#4286,#1311,.T.);
#5545=EDGE_CURVE('',#4287,#4288,#1312,.T.);
#5546=EDGE_CURVE('',#4288,#4281,#1313,.T.);
#5547=EDGE_CURVE('',#4280,#4283,#1314,.T.);
#5548=EDGE_CURVE('',#4279,#4284,#1315,.T.);
#5549=EDGE_CURVE('',#4285,#4240,#1316,.T.);
#5550=EDGE_CURVE('',#4289,#4287,#1317,.T.);
#5551=EDGE_CURVE('',#4289,#4263,#1318,.T.);
#5552=EDGE_CURVE('',#4288,#4262,#1319,.T.);
#5553=EDGE_CURVE('',#4290,#4239,#1320,.T.);
#5554=EDGE_CURVE('',#4290,#4286,#1321,.T.);
#5555=EDGE_CURVE('',#4289,#4290,#1322,.T.);
#5556=EDGE_CURVE('',#4248,#4258,#481,.T.);
#5557=EDGE_CURVE('',#4249,#4256,#482,.T.);
#5558=EDGE_CURVE('',#4278,#4250,#483,.T.);
#5559=EDGE_CURVE('',#4259,#4247,#484,.T.);
#5560=EDGE_CURVE('',#4257,#4246,#485,.T.);
#5561=EDGE_CURVE('',#4245,#4275,#486,.T.);
#5562=EDGE_CURVE('',#4291,#4277,#1323,.T.);
#5563=EDGE_CURVE('',#4273,#4291,#3456,.T.);
#5564=EDGE_CURVE('',#4237,#4253,#487,.T.);
#5565=EDGE_CURVE('',#4292,#4291,#3457,.T.);
#5566=EDGE_CURVE('',#4274,#4292,#3458,.T.);
#5567=EDGE_CURVE('',#4238,#4292,#1324,.T.);
#5568=EDGE_CURVE('',#4293,#4272,#3459,.T.);
#5569=EDGE_CURVE('',#4276,#4293,#1325,.T.);
#5570=EDGE_CURVE('',#4242,#4265,#488,.T.);
#5571=EDGE_CURVE('',#4294,#4271,#3460,.T.);
#5572=EDGE_CURVE('',#4293,#4294,#3461,.T.);
#5573=EDGE_CURVE('',#4294,#4264,#1326,.T.);
#5574=EDGE_CURVE('',#4276,#4264,#1327,.T.);
#5575=EDGE_CURVE('',#4277,#4238,#1328,.T.);
#7789=ORIENTED_EDGE('',*,*,#5420,.F.);
#7790=ORIENTED_EDGE('',*,*,#5421,.F.);
#7791=ORIENTED_EDGE('',*,*,#5422,.F.);
#7792=ORIENTED_EDGE('',*,*,#5423,.F.);
#7793=ORIENTED_EDGE('',*,*,#5424,.F.);
#7794=ORIENTED_EDGE('',*,*,#5425,.F.);
#7795=ORIENTED_EDGE('',*,*,#5426,.F.);
#7796=ORIENTED_EDGE('',*,*,#5427,.F.);
#7797=ORIENTED_EDGE('',*,*,#5428,.F.);
#7798=ORIENTED_EDGE('',*,*,#5429,.F.);
#7799=ORIENTED_EDGE('',*,*,#5430,.F.);
#7800=ORIENTED_EDGE('',*,*,#5431,.F.);
#7801=ORIENTED_EDGE('',*,*,#5432,.F.);
#7802=ORIENTED_EDGE('',*,*,#5433,.F.);
#7803=ORIENTED_EDGE('',*,*,#5434,.F.);
#7804=ORIENTED_EDGE('',*,*,#5435,.F.);
#7805=ORIENTED_EDGE('',*,*,#5436,.F.);
#7806=ORIENTED_EDGE('',*,*,#5437,.F.);
#7807=ORIENTED_EDGE('',*,*,#5438,.T.);
#7808=ORIENTED_EDGE('',*,*,#5439,.F.);
#7809=ORIENTED_EDGE('',*,*,#5440,.F.);
#7810=ORIENTED_EDGE('',*,*,#5441,.F.);
#7811=ORIENTED_EDGE('',*,*,#5442,.T.);
#7812=ORIENTED_EDGE('',*,*,#5443,.T.);
#7813=ORIENTED_EDGE('',*,*,#5444,.F.);
#7814=ORIENTED_EDGE('',*,*,#5443,.F.);
#7815=ORIENTED_EDGE('',*,*,#5445,.T.);
#7816=ORIENTED_EDGE('',*,*,#5446,.T.);
#7817=ORIENTED_EDGE('',*,*,#5447,.F.);
#7818=ORIENTED_EDGE('',*,*,#5446,.F.);
#7819=ORIENTED_EDGE('',*,*,#5448,.T.);
#7820=ORIENTED_EDGE('',*,*,#5449,.T.);
#7821=ORIENTED_EDGE('',*,*,#5450,.F.);
#7822=ORIENTED_EDGE('',*,*,#5449,.F.);
#7823=ORIENTED_EDGE('',*,*,#5420,.T.);
#7824=ORIENTED_EDGE('',*,*,#5451,.T.);
#7825=ORIENTED_EDGE('',*,*,#5452,.T.);
#7826=ORIENTED_EDGE('',*,*,#5453,.F.);
#7827=ORIENTED_EDGE('',*,*,#5454,.T.);
#7828=ORIENTED_EDGE('',*,*,#5455,.T.);
#7829=ORIENTED_EDGE('',*,*,#5456,.F.);
#7830=ORIENTED_EDGE('',*,*,#5455,.F.);
#7831=ORIENTED_EDGE('',*,*,#5457,.F.);
#7832=ORIENTED_EDGE('',*,*,#5458,.T.);
#7833=ORIENTED_EDGE('',*,*,#5459,.F.);
#7834=ORIENTED_EDGE('',*,*,#5458,.F.);
#7835=ORIENTED_EDGE('',*,*,#5460,.T.);
#7836=ORIENTED_EDGE('',*,*,#5461,.T.);
#7837=ORIENTED_EDGE('',*,*,#5462,.F.);
#7838=ORIENTED_EDGE('',*,*,#5461,.F.);
#7839=ORIENTED_EDGE('',*,*,#5463,.F.);
#7840=ORIENTED_EDGE('',*,*,#5464,.T.);
#7841=ORIENTED_EDGE('',*,*,#5427,.T.);
#7842=ORIENTED_EDGE('',*,*,#5465,.F.);
#7843=ORIENTED_EDGE('',*,*,#5432,.T.);
#7844=ORIENTED_EDGE('',*,*,#5466,.T.);
#7845=ORIENTED_EDGE('',*,*,#5434,.T.);
#7846=ORIENTED_EDGE('',*,*,#5467,.F.);
#7847=ORIENTED_EDGE('',*,*,#5468,.T.);
#7848=ORIENTED_EDGE('',*,*,#5428,.T.);
#7849=ORIENTED_EDGE('',*,*,#5464,.F.);
#7850=ORIENTED_EDGE('',*,*,#5469,.F.);
#7851=ORIENTED_EDGE('',*,*,#5470,.T.);
#7852=ORIENTED_EDGE('',*,*,#5471,.T.);
#7853=ORIENTED_EDGE('',*,*,#5451,.F.);
#7854=ORIENTED_EDGE('',*,*,#5424,.T.);
#7855=ORIENTED_EDGE('',*,*,#5465,.T.);
#7856=ORIENTED_EDGE('',*,*,#5472,.T.);
#7857=ORIENTED_EDGE('',*,*,#5473,.F.);
#7858=ORIENTED_EDGE('',*,*,#5474,.F.);
#7859=ORIENTED_EDGE('',*,*,#5475,.T.);
#7860=ORIENTED_EDGE('',*,*,#5476,.T.);
#7861=ORIENTED_EDGE('',*,*,#5477,.F.);
#7862=ORIENTED_EDGE('',*,*,#5478,.F.);
#7863=ORIENTED_EDGE('',*,*,#5479,.F.);
#7864=ORIENTED_EDGE('',*,*,#5473,.T.);
#7865=ORIENTED_EDGE('',*,*,#5480,.T.);
#7866=ORIENTED_EDGE('',*,*,#5430,.T.);
#7867=ORIENTED_EDGE('',*,*,#5481,.T.);
#7868=ORIENTED_EDGE('',*,*,#5422,.T.);
#7869=ORIENTED_EDGE('',*,*,#5482,.T.);
#7870=ORIENTED_EDGE('',*,*,#5483,.T.);
#7871=ORIENTED_EDGE('',*,*,#5484,.T.);
#7872=ORIENTED_EDGE('',*,*,#5485,.T.);
#7873=ORIENTED_EDGE('',*,*,#5486,.T.);
#7874=ORIENTED_EDGE('',*,*,#5487,.T.);
#7875=ORIENTED_EDGE('',*,*,#5488,.T.);
#7876=ORIENTED_EDGE('',*,*,#5448,.F.);
#7877=ORIENTED_EDGE('',*,*,#5444,.T.);
#7878=ORIENTED_EDGE('',*,*,#5489,.F.);
#7879=ORIENTED_EDGE('',*,*,#5436,.T.);
#7880=ORIENTED_EDGE('',*,*,#5490,.T.);
#7881=ORIENTED_EDGE('',*,*,#5491,.T.);
#7882=ORIENTED_EDGE('',*,*,#5492,.T.);
#7883=ORIENTED_EDGE('',*,*,#5493,.T.);
#7884=ORIENTED_EDGE('',*,*,#5494,.F.);
#7885=ORIENTED_EDGE('',*,*,#5495,.T.);
#7886=ORIENTED_EDGE('',*,*,#5496,.T.);
#7887=ORIENTED_EDGE('',*,*,#5425,.T.);
#7888=ORIENTED_EDGE('',*,*,#5454,.F.);
#7889=ORIENTED_EDGE('',*,*,#5462,.T.);
#7890=ORIENTED_EDGE('',*,*,#5497,.T.);
#7891=ORIENTED_EDGE('',*,*,#5498,.T.);
#7892=ORIENTED_EDGE('',*,*,#5499,.F.);
#7893=ORIENTED_EDGE('',*,*,#5500,.T.);
#7894=ORIENTED_EDGE('',*,*,#5499,.T.);
#7895=ORIENTED_EDGE('',*,*,#5501,.T.);
#7896=ORIENTED_EDGE('',*,*,#5502,.F.);
#7897=ORIENTED_EDGE('',*,*,#5503,.T.);
#7898=ORIENTED_EDGE('',*,*,#5502,.T.);
#7899=ORIENTED_EDGE('',*,*,#5504,.T.);
#7900=ORIENTED_EDGE('',*,*,#5466,.F.);
#7901=ORIENTED_EDGE('',*,*,#5505,.T.);
#7902=ORIENTED_EDGE('',*,*,#5506,.F.);
#7903=ORIENTED_EDGE('',*,*,#5507,.T.);
#7904=ORIENTED_EDGE('',*,*,#5453,.T.);
#7905=ORIENTED_EDGE('',*,*,#5508,.T.);
#7906=ORIENTED_EDGE('',*,*,#5509,.T.);
#7907=ORIENTED_EDGE('',*,*,#5510,.T.);
#7908=ORIENTED_EDGE('',*,*,#5511,.T.);
#7909=ORIENTED_EDGE('',*,*,#5512,.T.);
#7910=ORIENTED_EDGE('',*,*,#5506,.T.);
#7911=ORIENTED_EDGE('',*,*,#5513,.T.);
#7912=ORIENTED_EDGE('',*,*,#5514,.F.);
#7913=ORIENTED_EDGE('',*,*,#5515,.T.);
#7914=ORIENTED_EDGE('',*,*,#5516,.T.);
#7915=ORIENTED_EDGE('',*,*,#5494,.T.);
#7916=ORIENTED_EDGE('',*,*,#5517,.T.);
#7917=ORIENTED_EDGE('',*,*,#5518,.T.);
#7918=ORIENTED_EDGE('',*,*,#5519,.T.);
#7919=ORIENTED_EDGE('',*,*,#5520,.T.);
#7920=ORIENTED_EDGE('',*,*,#5521,.T.);
#7921=ORIENTED_EDGE('',*,*,#5445,.F.);
#7922=ORIENTED_EDGE('',*,*,#5522,.T.);
#7923=ORIENTED_EDGE('',*,*,#5523,.T.);
#7924=ORIENTED_EDGE('',*,*,#5515,.F.);
#7925=ORIENTED_EDGE('',*,*,#5524,.T.);
#7926=ORIENTED_EDGE('',*,*,#5459,.T.);
#7927=ORIENTED_EDGE('',*,*,#5484,.F.);
#7928=ORIENTED_EDGE('',*,*,#5525,.T.);
#7929=ORIENTED_EDGE('',*,*,#5518,.F.);
#7930=ORIENTED_EDGE('',*,*,#5526,.T.);
#7931=ORIENTED_EDGE('',*,*,#5527,.T.);
#7932=ORIENTED_EDGE('',*,*,#5528,.T.);
#7933=ORIENTED_EDGE('',*,*,#5529,.T.);
#7934=ORIENTED_EDGE('',*,*,#5530,.T.);
#7935=ORIENTED_EDGE('',*,*,#5497,.F.);
#7936=ORIENTED_EDGE('',*,*,#5531,.T.);
#7937=ORIENTED_EDGE('',*,*,#5532,.F.);
#7938=ORIENTED_EDGE('',*,*,#5438,.F.);
#7939=ORIENTED_EDGE('',*,*,#5533,.F.);
#7940=ORIENTED_EDGE('',*,*,#5534,.F.);
#7941=ORIENTED_EDGE('',*,*,#5535,.F.);
#7942=ORIENTED_EDGE('',*,*,#5536,.F.);
#7943=ORIENTED_EDGE('',*,*,#5513,.F.);
#7944=ORIENTED_EDGE('',*,*,#5508,.F.);
#7945=ORIENTED_EDGE('',*,*,#5452,.F.);
#7946=ORIENTED_EDGE('',*,*,#5471,.F.);
#7947=ORIENTED_EDGE('',*,*,#5442,.F.);
#7948=ORIENTED_EDGE('',*,*,#5450,.T.);
#7949=ORIENTED_EDGE('',*,*,#5440,.T.);
#7950=ORIENTED_EDGE('',*,*,#5537,.T.);
#7951=ORIENTED_EDGE('',*,*,#5469,.T.);
#7952=ORIENTED_EDGE('',*,*,#5463,.T.);
#7953=ORIENTED_EDGE('',*,*,#5474,.T.);
#7954=ORIENTED_EDGE('',*,*,#5479,.T.);
#7955=ORIENTED_EDGE('',*,*,#5538,.T.);
#7956=ORIENTED_EDGE('',*,*,#5539,.T.);
#7957=ORIENTED_EDGE('',*,*,#5540,.T.);
#7958=ORIENTED_EDGE('',*,*,#5541,.T.);
#7959=ORIENTED_EDGE('',*,*,#5460,.F.);
#7960=ORIENTED_EDGE('',*,*,#5456,.T.);
#7961=ORIENTED_EDGE('',*,*,#5539,.F.);
#7962=ORIENTED_EDGE('',*,*,#5542,.T.);
#7963=ORIENTED_EDGE('',*,*,#5543,.F.);
#7964=ORIENTED_EDGE('',*,*,#5544,.F.);
#7965=ORIENTED_EDGE('',*,*,#5545,.T.);
#7966=ORIENTED_EDGE('',*,*,#5546,.T.);
#7967=ORIENTED_EDGE('',*,*,#5535,.T.);
#7968=ORIENTED_EDGE('',*,*,#5547,.T.);
#7969=ORIENTED_EDGE('',*,*,#5540,.F.);
#7970=ORIENTED_EDGE('',*,*,#5547,.F.);
#7971=ORIENTED_EDGE('',*,*,#5534,.T.);
#7972=ORIENTED_EDGE('',*,*,#5548,.T.);
#7973=ORIENTED_EDGE('',*,*,#5541,.F.);
#7974=ORIENTED_EDGE('',*,*,#5548,.F.);
#7975=ORIENTED_EDGE('',*,*,#5533,.T.);
#7976=ORIENTED_EDGE('',*,*,#5441,.T.);
#7977=ORIENTED_EDGE('',*,*,#5478,.T.);
#7978=ORIENTED_EDGE('',*,*,#5549,.F.);
#7979=ORIENTED_EDGE('',*,*,#5542,.F.);
#7980=ORIENTED_EDGE('',*,*,#5538,.F.);
#7981=ORIENTED_EDGE('',*,*,#5550,.F.);
#7982=ORIENTED_EDGE('',*,*,#5551,.T.);
#7983=ORIENTED_EDGE('',*,*,#5509,.F.);
#7984=ORIENTED_EDGE('',*,*,#5552,.F.);
#7985=ORIENTED_EDGE('',*,*,#5545,.F.);
#7986=ORIENTED_EDGE('',*,*,#5553,.F.);
#7987=ORIENTED_EDGE('',*,*,#5554,.T.);
#7988=ORIENTED_EDGE('',*,*,#5543,.T.);
#7989=ORIENTED_EDGE('',*,*,#5549,.T.);
#7990=ORIENTED_EDGE('',*,*,#5477,.T.);
#7991=ORIENTED_EDGE('',*,*,#5536,.T.);
#7992=ORIENTED_EDGE('',*,*,#5546,.F.);
#7993=ORIENTED_EDGE('',*,*,#5552,.T.);
#7994=ORIENTED_EDGE('',*,*,#5514,.T.);
#7995=ORIENTED_EDGE('',*,*,#5555,.F.);
#7996=ORIENTED_EDGE('',*,*,#5550,.T.);
#7997=ORIENTED_EDGE('',*,*,#5544,.T.);
#7998=ORIENTED_EDGE('',*,*,#5554,.F.);
#7999=ORIENTED_EDGE('',*,*,#5491,.F.);
#8000=ORIENTED_EDGE('',*,*,#5556,.T.);
#8001=ORIENTED_EDGE('',*,*,#5501,.F.);
#8002=ORIENTED_EDGE('',*,*,#5557,.F.);
#8003=ORIENTED_EDGE('',*,*,#5530,.F.);
#8004=ORIENTED_EDGE('',*,*,#5558,.T.);
#8005=ORIENTED_EDGE('',*,*,#5492,.F.);
#8006=ORIENTED_EDGE('',*,*,#5557,.T.);
#8007=ORIENTED_EDGE('',*,*,#5498,.F.);
#8008=ORIENTED_EDGE('',*,*,#5503,.F.);
#8009=ORIENTED_EDGE('',*,*,#5559,.T.);
#8010=ORIENTED_EDGE('',*,*,#5487,.F.);
#8011=ORIENTED_EDGE('',*,*,#5560,.F.);
#8012=ORIENTED_EDGE('',*,*,#5531,.F.);
#8013=ORIENTED_EDGE('',*,*,#5500,.F.);
#8014=ORIENTED_EDGE('',*,*,#5560,.T.);
#8015=ORIENTED_EDGE('',*,*,#5486,.F.);
#8016=ORIENTED_EDGE('',*,*,#5561,.T.);
#8017=ORIENTED_EDGE('',*,*,#5556,.F.);
#8018=ORIENTED_EDGE('',*,*,#5490,.F.);
#8019=ORIENTED_EDGE('',*,*,#5435,.T.);
#8020=ORIENTED_EDGE('',*,*,#5504,.F.);
#8021=ORIENTED_EDGE('',*,*,#5559,.F.);
#8022=ORIENTED_EDGE('',*,*,#5505,.F.);
#8023=ORIENTED_EDGE('',*,*,#5431,.T.);
#8024=ORIENTED_EDGE('',*,*,#5488,.F.);
#8025=ORIENTED_EDGE('',*,*,#5558,.F.);
#8026=ORIENTED_EDGE('',*,*,#5529,.F.);
#8027=ORIENTED_EDGE('',*,*,#5562,.F.);
#8028=ORIENTED_EDGE('',*,*,#5563,.F.);
#8029=ORIENTED_EDGE('',*,*,#5524,.F.);
#8030=ORIENTED_EDGE('',*,*,#5517,.F.);
#8031=ORIENTED_EDGE('',*,*,#5493,.F.);
#8032=ORIENTED_EDGE('',*,*,#5426,.T.);
#8033=ORIENTED_EDGE('',*,*,#5496,.F.);
#8034=ORIENTED_EDGE('',*,*,#5564,.F.);
#8035=ORIENTED_EDGE('',*,*,#5480,.F.);
#8036=ORIENTED_EDGE('',*,*,#5472,.F.);
#8037=ORIENTED_EDGE('',*,*,#5563,.T.);
#8038=ORIENTED_EDGE('',*,*,#5565,.F.);
#8039=ORIENTED_EDGE('',*,*,#5566,.F.);
#8040=ORIENTED_EDGE('',*,*,#5522,.F.);
#8041=ORIENTED_EDGE('',*,*,#5516,.F.);
#8042=ORIENTED_EDGE('',*,*,#5523,.F.);
#8043=ORIENTED_EDGE('',*,*,#5566,.T.);
#8044=ORIENTED_EDGE('',*,*,#5567,.F.);
#8045=ORIENTED_EDGE('',*,*,#5475,.F.);
#8046=ORIENTED_EDGE('',*,*,#5564,.T.);
#8047=ORIENTED_EDGE('',*,*,#5495,.F.);
#8048=ORIENTED_EDGE('',*,*,#5526,.F.);
#8049=ORIENTED_EDGE('',*,*,#5521,.F.);
#8050=ORIENTED_EDGE('',*,*,#5568,.F.);
#8051=ORIENTED_EDGE('',*,*,#5569,.F.);
#8052=ORIENTED_EDGE('',*,*,#5527,.F.);
#8053=ORIENTED_EDGE('',*,*,#5561,.F.);
#8054=ORIENTED_EDGE('',*,*,#5485,.F.);
#8055=ORIENTED_EDGE('',*,*,#5507,.F.);
#8056=ORIENTED_EDGE('',*,*,#5512,.F.);
#8057=ORIENTED_EDGE('',*,*,#5570,.F.);
#8058=ORIENTED_EDGE('',*,*,#5482,.F.);
#8059=ORIENTED_EDGE('',*,*,#5421,.T.);
#8060=ORIENTED_EDGE('',*,*,#5568,.T.);
#8061=ORIENTED_EDGE('',*,*,#5520,.F.);
#8062=ORIENTED_EDGE('',*,*,#5571,.F.);
#8063=ORIENTED_EDGE('',*,*,#5572,.F.);
#8064=ORIENTED_EDGE('',*,*,#5570,.T.);
#8065=ORIENTED_EDGE('',*,*,#5511,.F.);
#8066=ORIENTED_EDGE('',*,*,#5573,.F.);
#8067=ORIENTED_EDGE('',*,*,#5571,.T.);
#8068=ORIENTED_EDGE('',*,*,#5519,.F.);
#8069=ORIENTED_EDGE('',*,*,#5525,.F.);
#8070=ORIENTED_EDGE('',*,*,#5483,.F.);
#8071=ORIENTED_EDGE('',*,*,#5439,.T.);
#8072=ORIENTED_EDGE('',*,*,#5532,.T.);
#8073=ORIENTED_EDGE('',*,*,#5470,.F.);
#8074=ORIENTED_EDGE('',*,*,#5423,.T.);
#8075=ORIENTED_EDGE('',*,*,#5481,.F.);
#8076=ORIENTED_EDGE('',*,*,#5433,.T.);
#8077=ORIENTED_EDGE('',*,*,#5467,.T.);
#8078=ORIENTED_EDGE('',*,*,#5437,.T.);
#8079=ORIENTED_EDGE('',*,*,#5489,.T.);
#8080=ORIENTED_EDGE('',*,*,#5429,.T.);
#8081=ORIENTED_EDGE('',*,*,#5468,.F.);
#8082=ORIENTED_EDGE('',*,*,#5537,.F.);
#8083=ORIENTED_EDGE('',*,*,#5574,.T.);
#8084=ORIENTED_EDGE('',*,*,#5510,.F.);
#8085=ORIENTED_EDGE('',*,*,#5551,.F.);
#8086=ORIENTED_EDGE('',*,*,#5555,.T.);
#8087=ORIENTED_EDGE('',*,*,#5553,.T.);
#8088=ORIENTED_EDGE('',*,*,#5476,.F.);
#8089=ORIENTED_EDGE('',*,*,#5575,.F.);
#8090=ORIENTED_EDGE('',*,*,#5528,.F.);
#8091=ORIENTED_EDGE('',*,*,#5562,.T.);
#8092=ORIENTED_EDGE('',*,*,#5575,.T.);
#8093=ORIENTED_EDGE('',*,*,#5567,.T.);
#8094=ORIENTED_EDGE('',*,*,#5565,.T.);
#8095=ORIENTED_EDGE('',*,*,#5457,.T.);
#8096=ORIENTED_EDGE('',*,*,#5569,.T.);
#8097=ORIENTED_EDGE('',*,*,#5572,.T.);
#8098=ORIENTED_EDGE('',*,*,#5573,.T.);
#8099=ORIENTED_EDGE('',*,*,#5574,.F.);
#8100=ORIENTED_EDGE('',*,*,#5447,.T.);
#8800=ADVANCED_FACE('',(#2450),#652,.T.);
#8801=ADVANCED_FACE('',(#2451),#653,.T.);
#8802=ADVANCED_FACE('',(#2452),#654,.T.);
#8803=ADVANCED_FACE('',(#2453),#655,.T.);
#8804=ADVANCED_FACE('',(#2454),#2017,.F.);
#8805=ADVANCED_FACE('',(#2455),#2018,.F.);
#8806=ADVANCED_FACE('',(#2456),#2019,.F.);
#8807=ADVANCED_FACE('',(#2457),#2020,.F.);
#8808=ADVANCED_FACE('',(#2458),#2021,.F.);
#8809=ADVANCED_FACE('',(#2459),#2022,.F.);
#8810=ADVANCED_FACE('',(#2460),#2023,.F.);
#8811=ADVANCED_FACE('',(#2461),#2024,.F.);
#8812=ADVANCED_FACE('',(#2462),#2025,.F.);
#8813=ADVANCED_FACE('',(#2463),#2026,.T.);
#8814=ADVANCED_FACE('',(#2464),#842,.F.);
#8815=ADVANCED_FACE('',(#2465),#843,.F.);
#8816=ADVANCED_FACE('',(#2466),#844,.F.);
#8817=ADVANCED_FACE('',(#2467),#845,.F.);
#8818=ADVANCED_FACE('',(#2468,#737,#738),#846,.F.);
#8819=ADVANCED_FACE('',(#2469,#739,#740),#847,.T.);
#8820=ADVANCED_FACE('',(#2470),#848,.F.);
#8821=ADVANCED_FACE('',(#2471),#2027,.F.);
#8822=ADVANCED_FACE('',(#2472),#849,.F.);
#8823=ADVANCED_FACE('',(#2473),#850,.F.);
#8824=ADVANCED_FACE('',(#2474),#851,.F.);
#8825=ADVANCED_FACE('',(#2475),#852,.T.);
#8826=ADVANCED_FACE('',(#2476,#741),#853,.T.);
#8827=ADVANCED_FACE('',(#2477,#742),#854,.F.);
#8828=ADVANCED_FACE('',(#2478),#855,.T.);
#8829=ADVANCED_FACE('',(#2479),#856,.F.);
#8830=ADVANCED_FACE('',(#2480,#743,#744),#857,.T.);
#8831=ADVANCED_FACE('',(#2481,#745,#746),#858,.F.);
#8832=ADVANCED_FACE('',(#2482),#859,.T.);
#8833=ADVANCED_FACE('',(#2483),#2028,.T.);
#8834=ADVANCED_FACE('',(#2484),#860,.T.);
#8835=ADVANCED_FACE('',(#2485),#861,.F.);
#8836=ADVANCED_FACE('',(#2486),#862,.F.);
#8837=ADVANCED_FACE('',(#2487),#863,.T.);
#8838=ADVANCED_FACE('',(#2488),#864,.F.);
#8839=ADVANCED_FACE('',(#2489),#865,.T.);
#8840=ADVANCED_FACE('',(#2490),#656,.T.);
#8841=ADVANCED_FACE('',(#2491),#2029,.T.);
#8842=ADVANCED_FACE('',(#2492),#657,.T.);
#8843=ADVANCED_FACE('',(#2493),#2030,.T.);
#8844=ADVANCED_FACE('',(#2494),#2031,.T.);
#8845=ADVANCED_FACE('',(#2495),#2032,.T.);
#8846=ADVANCED_FACE('',(#2496),#2033,.T.);
#8847=ADVANCED_FACE('',(#2497),#2034,.T.);
#8848=ADVANCED_FACE('',(#2498),#658,.T.);
#8849=ADVANCED_FACE('',(#2499),#2035,.T.);
#8850=ADVANCED_FACE('',(#2500),#2036,.T.);
#8851=ADVANCED_FACE('',(#2501),#2037,.T.);
#8852=ADVANCED_FACE('',(#2502),#659,.T.);
#8853=ADVANCED_FACE('',(#2503),#2038,.T.);
#8854=ADVANCED_FACE('',(#2504),#2039,.T.);
#8855=ADVANCED_FACE('',(#2505),#866,.F.);
#8856=ADVANCED_FACE('',(#2506,#747),#867,.F.);
#8857=ADVANCED_FACE('',(#2507,#748),#868,.F.);
#8932=CLOSED_SHELL('',(#8800,#8801,#8802,#8803,#8804,#8805,#8806,#8807,
#8808,#8809,#8810,#8811,#8812,#8813,#8814,#8815,#8816,#8817,#8818,#8819,
#8820,#8821,#8822,#8823,#8824,#8825,#8826,#8827,#8828,#8829,#8830,#8831,
#8832,#8833,#8834,#8835,#8836,#8837,#8838,#8839,#8840,#8841,#8842,#8843,
#8844,#8845,#8846,#8847,#8848,#8849,#8850,#8851,#8852,#8853,#8854,#8855,
#8856,#8857));
#9703=AXIS2_PLACEMENT_3D('',#45245,#11580,#11581);
#9704=AXIS2_PLACEMENT_3D('',#45246,#11582,#11583);
#9705=AXIS2_PLACEMENT_3D('',#45249,#11584,#11585);
#9706=AXIS2_PLACEMENT_3D('',#45266,#11586,#11587);
#9707=AXIS2_PLACEMENT_3D('',#45288,#11588,#11589);
#9708=AXIS2_PLACEMENT_3D('',#45291,#11590,#11591);
#9709=AXIS2_PLACEMENT_3D('',#45308,#11592,#11593);
#9710=AXIS2_PLACEMENT_3D('',#45332,#11594,#11595);
#9711=AXIS2_PLACEMENT_3D('',#45335,#11596,#11597);
#9712=AXIS2_PLACEMENT_3D('',#45360,#11598,#11599);
#9713=AXIS2_PLACEMENT_3D('',#45377,#11600,#11601);
#9714=AXIS2_PLACEMENT_3D('',#45380,#11602,#11603);
#9715=AXIS2_PLACEMENT_3D('',#45405,#11604,#11605);
#9716=AXIS2_PLACEMENT_3D('',#45422,#11606,#11607);
#9717=AXIS2_PLACEMENT_3D('',#45425,#11608,#11609);
#9718=AXIS2_PLACEMENT_3D('',#45429,#11611,#11612);
#9719=AXIS2_PLACEMENT_3D('',#45431,#11614,#11615);
#9720=AXIS2_PLACEMENT_3D('',#45433,#11616,#11617);
#9721=AXIS2_PLACEMENT_3D('',#45436,#11619,#11620);
#9722=AXIS2_PLACEMENT_3D('',#45437,#11621,#11622);
#9723=AXIS2_PLACEMENT_3D('',#45439,#11623,#11624);
#9724=AXIS2_PLACEMENT_3D('',#45442,#11626,#11627);
#9725=AXIS2_PLACEMENT_3D('',#45443,#11628,#11629);
#9726=AXIS2_PLACEMENT_3D('',#45445,#11630,#11631);
#9727=AXIS2_PLACEMENT_3D('',#45448,#11633,#11634);
#9728=AXIS2_PLACEMENT_3D('',#45449,#11635,#11636);
#9729=AXIS2_PLACEMENT_3D('',#45453,#11638,#11639);
#9730=AXIS2_PLACEMENT_3D('',#45455,#11641,#11642);
#9731=AXIS2_PLACEMENT_3D('',#45457,#11643,#11644);
#9732=AXIS2_PLACEMENT_3D('',#45460,#11646,#11647);
#9733=AXIS2_PLACEMENT_3D('',#45461,#11648,#11649);
#9734=AXIS2_PLACEMENT_3D('',#45463,#11650,#11651);
#9735=AXIS2_PLACEMENT_3D('',#45466,#11653,#11654);
#9736=AXIS2_PLACEMENT_3D('',#45467,#11655,#11656);
#9737=AXIS2_PLACEMENT_3D('',#45469,#11657,#11658);
#9738=AXIS2_PLACEMENT_3D('',#45472,#11660,#11661);
#9739=AXIS2_PLACEMENT_3D('',#45473,#11662,#11663);
#9740=AXIS2_PLACEMENT_3D('',#45476,#11664,#11665);
#9741=AXIS2_PLACEMENT_3D('',#45479,#11668,#11669);
#9742=AXIS2_PLACEMENT_3D('',#45482,#11672,#11673);
#9743=AXIS2_PLACEMENT_3D('',#45486,#11676,#11677);
#9744=AXIS2_PLACEMENT_3D('',#45490,#11680,#11681);
#9745=AXIS2_PLACEMENT_3D('',#45496,#11685,#11686);
#9746=AXIS2_PLACEMENT_3D('',#45507,#11692,#11693);
#9747=AXIS2_PLACEMENT_3D('',#45508,#11694,#11695);
#9748=AXIS2_PLACEMENT_3D('',#45509,#11696,#11697);
#9749=AXIS2_PLACEMENT_3D('',#45521,#11703,#11704);
#9750=AXIS2_PLACEMENT_3D('',#45523,#11706,#11707);
#9751=AXIS2_PLACEMENT_3D('',#45524,#11708,#11709);
#9752=AXIS2_PLACEMENT_3D('',#45528,#11711,#11712);
#9753=AXIS2_PLACEMENT_3D('',#45538,#11718,#11719);
#9754=AXIS2_PLACEMENT_3D('',#45547,#11724,#11725);
#9755=AXIS2_PLACEMENT_3D('',#45549,#11726,#11727);
#9756=AXIS2_PLACEMENT_3D('',#45552,#11729,#11730);
#9757=AXIS2_PLACEMENT_3D('',#45553,#11731,#11732);
#9758=AXIS2_PLACEMENT_3D('',#45556,#11735,#11736);
#9759=AXIS2_PLACEMENT_3D('',#45562,#11740,#11741);
#9760=AXIS2_PLACEMENT_3D('',#45570,#11745,#11746);
#9761=AXIS2_PLACEMENT_3D('',#45574,#11749,#11750);
#9762=AXIS2_PLACEMENT_3D('',#45578,#11752,#11753);
#9763=AXIS2_PLACEMENT_3D('',#45579,#11754,#11755);
#9764=AXIS2_PLACEMENT_3D('',#45580,#11756,#11757);
#9765=AXIS2_PLACEMENT_3D('',#45587,#11760,#11761);
#9766=AXIS2_PLACEMENT_3D('',#45589,#11763,#11764);
#9767=AXIS2_PLACEMENT_3D('',#45592,#11765,#11766);
#9768=AXIS2_PLACEMENT_3D('',#45595,#11769,#11770);
#9769=AXIS2_PLACEMENT_3D('',#45596,#11771,#11772);
#9770=AXIS2_PLACEMENT_3D('',#45597,#11773,#11774);
#9771=AXIS2_PLACEMENT_3D('',#45598,#11775,#11776);
#9772=AXIS2_PLACEMENT_3D('',#45606,#11780,#11781);
#9773=AXIS2_PLACEMENT_3D('',#45607,#11782,#11783);
#9774=AXIS2_PLACEMENT_3D('',#45608,#11784,#11785);
#9775=AXIS2_PLACEMENT_3D('',#45609,#11786,#11787);
#9776=AXIS2_PLACEMENT_3D('',#45613,#11789,#11790);
#9777=AXIS2_PLACEMENT_3D('',#45617,#11793,#11794);
#9778=AXIS2_PLACEMENT_3D('',#45618,#11795,#11796);
#9779=AXIS2_PLACEMENT_3D('',#45624,#11799,#11800);
#9780=AXIS2_PLACEMENT_3D('',#45626,#11802,#11803);
#9781=AXIS2_PLACEMENT_3D('',#45637,#11810,#11811);
#9782=AXIS2_PLACEMENT_3D('',#45639,#11813,#11814);
#9783=AXIS2_PLACEMENT_3D('',#45640,#11815,#11816);
#9784=AXIS2_PLACEMENT_3D('',#45642,#11818,#11819);
#9785=AXIS2_PLACEMENT_3D('',#45647,#11823,#11824);
#9786=AXIS2_PLACEMENT_3D('',#45651,#11827,#11828);
#9787=AXIS2_PLACEMENT_3D('',#45652,#11829,#11830);
#9788=AXIS2_PLACEMENT_3D('',#45654,#11832,#11833);
#9789=AXIS2_PLACEMENT_3D('',#45742,#11834,#11835);
#9790=AXIS2_PLACEMENT_3D('',#45751,#11836,#11837);
#9791=AXIS2_PLACEMENT_3D('',#45839,#11838,#11839);
#9792=AXIS2_PLACEMENT_3D('',#45848,#11840,#11841);
#9793=AXIS2_PLACEMENT_3D('',#45849,#11842,#11843);
#9794=AXIS2_PLACEMENT_3D('',#45850,#11844,#11845);
#9795=AXIS2_PLACEMENT_3D('',#45853,#11847,#11848);
#9796=AXIS2_PLACEMENT_3D('',#45854,#11849,#11850);
#9797=AXIS2_PLACEMENT_3D('',#45865,#11851,#11852);
#9798=AXIS2_PLACEMENT_3D('',#45867,#11853,#11854);
#9799=AXIS2_PLACEMENT_3D('',#45868,#11855,#11856);
#9800=AXIS2_PLACEMENT_3D('',#45869,#11857,#11858);
#9801=AXIS2_PLACEMENT_3D('',#45871,#11860,#11861);
#9802=AXIS2_PLACEMENT_3D('',#45873,#11862,#11863);
#9803=AXIS2_PLACEMENT_3D('',#45875,#11865,#11866);
#9804=AXIS2_PLACEMENT_3D('',#45886,#11867,#11868);
#9805=AXIS2_PLACEMENT_3D('',#45888,#11869,#11870);
#9806=AXIS2_PLACEMENT_3D('',#45889,#11871,#11872);
#9807=AXIS2_PLACEMENT_3D('',#45890,#11873,#11874);
#9808=AXIS2_PLACEMENT_3D('',#45892,#11876,#11877);
#9809=AXIS2_PLACEMENT_3D('',#45893,#11878,#11879);
#9810=AXIS2_PLACEMENT_3D('',#45896,#11882,#11883);
#9811=AXIS2_PLACEMENT_3D('',#45897,#11884,#11885);
#11580=DIRECTION('axis',(0.,0.,1.));
#11581=DIRECTION('refdir',(1.,0.,0.));
#11582=DIRECTION('center_axis',(4.00113358033595E-18,-1.90170940755474E-18,
-1.));
#11583=DIRECTION('ref_axis',(-0.925927934137781,0.377700226083253,0.));
#11584=DIRECTION('center_axis',(-4.00113358033595E-18,1.90170940755474E-18,
1.));
#11585=DIRECTION('ref_axis',(-0.925927934137781,0.377700226083253,-4.42303742342784E-18));
#11586=DIRECTION('center_axis',(4.00113358033595E-18,-1.90170940755474E-18,
-1.));
#11587=DIRECTION('ref_axis',(-0.925927934137781,0.377700226083253,-4.42303742342784E-18));
#11588=DIRECTION('center_axis',(4.00113358033595E-18,-1.90170940755474E-18,
-1.));
#11589=DIRECTION('ref_axis',(-0.925927934137781,0.377700226083253,0.));
#11590=DIRECTION('center_axis',(-4.00113358033595E-18,1.90170940755474E-18,
1.));
#11591=DIRECTION('ref_axis',(-0.925927934137781,0.377700226083253,-4.42303742342784E-18));
#11592=DIRECTION('center_axis',(4.00113358033595E-18,-1.90170940755474E-18,
-1.));
#11593=DIRECTION('ref_axis',(-0.925927934137781,0.377700226083253,-4.42303742342784E-18));
#11594=DIRECTION('center_axis',(4.00113358033595E-18,-1.90170940755474E-18,
-1.));
#11595=DIRECTION('ref_axis',(-0.925927934137781,0.377700226083253,0.));
#11596=DIRECTION('center_axis',(-4.00113358033595E-18,1.90170940755474E-18,
1.));
#11597=DIRECTION('ref_axis',(-0.925927934137781,0.377700226083253,-4.42303742342784E-18));
#11598=DIRECTION('center_axis',(4.00113358033595E-18,-1.90170940755474E-18,
-1.));
#11599=DIRECTION('ref_axis',(-0.925927934137781,0.377700226083253,-4.42303742342784E-18));
#11600=DIRECTION('center_axis',(4.00113358033595E-18,-1.90170940755474E-18,
-1.));
#11601=DIRECTION('ref_axis',(-0.925927934137781,0.377700226083253,0.));
#11602=DIRECTION('center_axis',(-4.00113358033595E-18,1.90170940755474E-18,
1.));
#11603=DIRECTION('ref_axis',(-0.925927934137781,0.377700226083253,-4.42303742342784E-18));
#11604=DIRECTION('center_axis',(4.00113358033595E-18,-1.90170940755474E-18,
-1.));
#11605=DIRECTION('ref_axis',(-0.925927934137781,0.377700226083253,-4.42303742342784E-18));
#11606=DIRECTION('center_axis',(4.00113358033595E-18,-1.90170940755474E-18,
-1.));
#11607=DIRECTION('ref_axis',(-0.925927934137781,0.377700226083253,-4.42303742342784E-18));
#11608=DIRECTION('center_axis',(-4.00113358033595E-18,1.90170940755474E-18,
1.));
#11609=DIRECTION('ref_axis',(-0.925927934137761,0.377700226083302,-4.42303742342785E-18));
#11610=DIRECTION('',(-4.00113358033595E-18,1.90170940755474E-18,1.));
#11611=DIRECTION('center_axis',(-4.00113358033595E-18,1.90170940755474E-18,
1.));
#11612=DIRECTION('ref_axis',(-0.925927934137761,0.377700226083302,-4.42303742342785E-18));
#11613=DIRECTION('',(4.00113358033595E-18,-1.90170940755474E-18,-1.));
#11614=DIRECTION('center_axis',(-4.00113358033595E-18,1.90170940755474E-18,
1.));
#11615=DIRECTION('ref_axis',(0.925927934137781,-0.377700226083254,4.42303742342784E-18));
#11616=DIRECTION('center_axis',(4.00113358033595E-18,-1.90170940755474E-18,
-1.));
#11617=DIRECTION('ref_axis',(-0.925927934137781,0.377700226083254,-4.42303742342784E-18));
#11618=DIRECTION('',(-4.00113358033595E-18,1.90170940755474E-18,1.));
#11619=DIRECTION('center_axis',(4.00113358033595E-18,-1.90170940755474E-18,
-1.));
#11620=DIRECTION('ref_axis',(-0.925927934137781,0.377700226083254,-4.42303742342784E-18));
#11621=DIRECTION('center_axis',(4.00113358033595E-18,-1.90170940755474E-18,
-1.));
#11622=DIRECTION('ref_axis',(-0.925927934137781,0.377700226083254,-4.42303742342784E-18));
#11623=DIRECTION('center_axis',(-4.00113358033595E-18,1.90170940755474E-18,
1.));
#11624=DIRECTION('ref_axis',(0.925927934137781,-0.377700226083254,4.42303742342784E-18));
#11625=DIRECTION('',(4.00113358033595E-18,-1.90170940755474E-18,-1.));
#11626=DIRECTION('center_axis',(-8.58733520598719E-17,-1.9880713026183E-16,
1.));
#11627=DIRECTION('ref_axis',(-0.377700226083251,-0.925927934137782,-2.16515459902737E-16));
#11628=DIRECTION('center_axis',(4.00113358033595E-18,-1.90170940755474E-18,
-1.));
#11629=DIRECTION('ref_axis',(-0.925927934137783,0.377700226083249,-4.42303742342784E-18));
#11630=DIRECTION('center_axis',(-4.00113358033595E-18,1.90170940755474E-18,
1.));
#11631=DIRECTION('ref_axis',(0.925927934137783,-0.377700226083249,4.42303742342784E-18));
#11632=DIRECTION('',(4.00113358033595E-18,-1.90170940755474E-18,-1.));
#11633=DIRECTION('center_axis',(-4.00113358033595E-18,1.90170940755474E-18,
1.));
#11634=DIRECTION('ref_axis',(-0.925927934137783,0.377700226083249,-4.42303742342784E-18));
#11635=DIRECTION('center_axis',(4.00113358033595E-18,-1.90170940755474E-18,
-1.));
#11636=DIRECTION('ref_axis',(-0.925927934137781,0.377700226083253,-4.42303742342784E-18));
#11637=DIRECTION('',(4.00113358033595E-18,-1.90170940755474E-18,-1.));
#11638=DIRECTION('center_axis',(4.00113358033595E-18,-1.90170940755474E-18,
-1.));
#11639=DIRECTION('ref_axis',(-0.925927934137781,0.377700226083253,-4.42303742342784E-18));
#11640=DIRECTION('',(4.00113358033595E-18,-1.90170940755474E-18,-1.));
#11641=DIRECTION('center_axis',(-4.00113358033595E-18,1.90170940755474E-18,
1.));
#11642=DIRECTION('ref_axis',(0.925927934137781,-0.377700226083254,4.42303742342784E-18));
#11643=DIRECTION('center_axis',(4.00113358033595E-18,-1.90170940755474E-18,
-1.));
#11644=DIRECTION('ref_axis',(-0.925927934137781,0.377700226083254,-4.42303742342784E-18));
#11645=DIRECTION('',(-4.00113358033595E-18,1.90170940755474E-18,1.));
#11646=DIRECTION('center_axis',(4.00113358033595E-18,-1.90170940755474E-18,
-1.));
#11647=DIRECTION('ref_axis',(-0.925927934137781,0.377700226083254,-4.42303742342784E-18));
#11648=DIRECTION('center_axis',(4.00113358033595E-18,-1.90170940755474E-18,
-1.));
#11649=DIRECTION('ref_axis',(-0.925927934137781,0.377700226083254,-4.42303742342784E-18));
#11650=DIRECTION('center_axis',(5.31244646680575E-17,1.18523594394076E-16,
-1.));
#11651=DIRECTION('ref_axis',(0.377700226083251,0.925927934137782,1.29809429219568E-16));
#11652=DIRECTION('',(4.00113358033595E-18,-1.90170940755474E-18,-1.));
#11653=DIRECTION('center_axis',(-4.00113358033595E-18,1.90170940755474E-18,
1.));
#11654=DIRECTION('ref_axis',(0.925927934137781,-0.377700226083254,4.42303742342784E-18));
#11655=DIRECTION('center_axis',(4.00113358033595E-18,-1.90170940755474E-18,
-1.));
#11656=DIRECTION('ref_axis',(-0.925927934137783,0.377700226083249,-4.42303742342784E-18));
#11657=DIRECTION('center_axis',(-4.00113358033595E-18,1.90170940755474E-18,
1.));
#11658=DIRECTION('ref_axis',(-0.925927934137783,0.377700226083249,-4.42303742342784E-18));
#11659=DIRECTION('',(4.00113358033595E-18,-1.90170940755474E-18,-1.));
#11660=DIRECTION('center_axis',(-4.00113358033595E-18,1.90170940755474E-18,
1.));
#11661=DIRECTION('ref_axis',(0.925927934137783,-0.377700226083249,4.42303742342784E-18));
#11662=DIRECTION('center_axis',(4.00113358033595E-18,-1.90170940755474E-18,
-1.));
#11663=DIRECTION('ref_axis',(-0.925927934137781,0.377700226083253,-4.42303742342784E-18));
#11664=DIRECTION('center_axis',(4.00113358033595E-18,-1.90170940755474E-18,
-1.));
#11665=DIRECTION('ref_axis',(-0.925927934137781,0.377700226083253,-4.42303742342784E-18));
#11666=DIRECTION('',(4.00113358033595E-18,-1.90170940755474E-18,-1.));
#11667=DIRECTION('',(4.00113358033595E-18,-1.90170940755474E-18,-1.));
#11668=DIRECTION('center_axis',(4.00113358033595E-18,-1.90170940755474E-18,
-1.));
#11669=DIRECTION('ref_axis',(-0.925927934137781,0.377700226083253,-4.42303742342784E-18));
#11670=DIRECTION('',(4.00113358033595E-18,-1.90170940755474E-18,-1.));
#11671=DIRECTION('',(4.00113358033595E-18,-1.90170940755474E-18,-1.));
#11672=DIRECTION('center_axis',(-0.925927934137781,0.377700226083253,-4.42303742342784E-18));
#11673=DIRECTION('ref_axis',(-4.00113358033595E-18,1.90170940755474E-18,
1.));
#11674=DIRECTION('',(4.00113358033595E-18,-1.90170940755474E-18,-1.));
#11675=DIRECTION('',(0.377700226083253,0.925927934137781,-2.49616805185364E-19));
#11676=DIRECTION('center_axis',(-0.925927934137781,0.377700226083253,-4.42303742342784E-18));
#11677=DIRECTION('ref_axis',(-4.00113358033595E-18,1.90170940755474E-18,
1.));
#11678=DIRECTION('',(4.00113358033595E-18,-1.90170940755474E-18,-1.));
#11679=DIRECTION('',(0.377700226083253,0.925927934137781,-2.49616805185364E-19));
#11680=DIRECTION('center_axis',(-0.925927934137781,0.377700226083253,-4.42303742342784E-18));
#11681=DIRECTION('ref_axis',(-0.377700226083253,-0.925927934137781,2.49616805185365E-19));
#11682=DIRECTION('',(0.377700226083253,0.925927934137781,-2.49616805185365E-19));
#11683=DIRECTION('',(4.00113358033595E-18,-1.90170940755474E-18,-1.));
#11684=DIRECTION('',(0.377700226083253,0.925927934137781,-2.49616805185365E-19));
#11685=DIRECTION('center_axis',(-0.999957006340362,0.00927283510161242,
-4.01859579470807E-18));
#11686=DIRECTION('ref_axis',(-0.00927283510161242,-0.999957006340362,1.86452579419776E-18));
#11687=DIRECTION('',(0.00927283510161242,0.999957006340362,-1.86452579419776E-18));
#11688=DIRECTION('',(-4.00113358033595E-18,1.90170940755474E-18,1.));
#11689=DIRECTION('',(0.00927283510161242,0.999957006340362,-1.86452579419776E-18));
#11690=DIRECTION('',(0.0087838870263115,0.947230192127013,-0.320433778574812));
#11691=DIRECTION('',(0.00927283510161242,0.999957006340362,-1.86452579419776E-18));
#11692=DIRECTION('center_axis',(0.999957006340363,-0.00927283510148195,
5.80621970068864E-14));
#11693=DIRECTION('ref_axis',(0.00927283510148195,0.999957006340363,-4.86701529800751E-12));
#11694=DIRECTION('center_axis',(4.00113358033595E-18,-1.90170940755474E-18,
-1.));
#11695=DIRECTION('ref_axis',(-0.925927934137781,0.377700226083253,-4.42303742342784E-18));
#11696=DIRECTION('center_axis',(-4.00113358033595E-18,1.90170940755474E-18,
1.));
#11697=DIRECTION('ref_axis',(-0.925927934137789,0.377700226083235,-4.42303742342784E-18));
#11698=DIRECTION('',(0.377700226083253,0.925927934137781,-2.49616805185365E-19));
#11699=DIRECTION('',(0.00927283510161242,0.999957006340362,-1.86452579419776E-18));
#11700=DIRECTION('',(-0.925927934137781,0.377700226083253,-4.42303742342784E-18));
#11701=DIRECTION('',(0.204644651309627,-0.978836332943542,2.68027284920621E-18));
#11702=DIRECTION('',(-0.377700226083253,-0.925927934137781,2.49616805185365E-19));
#11703=DIRECTION('center_axis',(4.00113358033595E-18,-1.90170940755474E-18,
-1.));
#11704=DIRECTION('ref_axis',(-0.925927934137781,0.377700226083253,-4.42303742342784E-18));
#11705=DIRECTION('',(-0.377700226083253,-0.925927934137781,2.49616805185364E-19));
#11706=DIRECTION('center_axis',(4.00113358033595E-18,-1.90170940755474E-18,
-1.));
#11707=DIRECTION('ref_axis',(-0.925927934137781,0.377700226083253,-4.42303742342784E-18));
#11708=DIRECTION('center_axis',(-4.00113358033595E-18,1.90170940755474E-18,
1.));
#11709=DIRECTION('ref_axis',(-0.925927934137781,0.377700226083255,-4.42303742342784E-18));
#11710=DIRECTION('',(0.377700226083253,0.925927934137781,-2.49616805185364E-19));
#11711=DIRECTION('center_axis',(-4.00113358033595E-18,1.90170940755474E-18,
1.));
#11712=DIRECTION('ref_axis',(-0.925927934137781,0.377700226083253,-4.42303742342784E-18));
#11713=DIRECTION('',(0.377700226083253,0.925927934137781,-2.49616805185365E-19));
#11714=DIRECTION('',(-0.204644651309627,0.978836332943542,-2.68027284920621E-18));
#11715=DIRECTION('',(-0.925927934137781,0.377700226083253,-4.42303742342784E-18));
#11716=DIRECTION('',(-0.00927283510161242,-0.999957006340362,1.86452579419776E-18));
#11717=DIRECTION('',(-0.377700226083253,-0.925927934137781,2.49616805185365E-19));
#11718=DIRECTION('center_axis',(0.925927934137782,-0.377700226083253,4.42303742342784E-18));
#11719=DIRECTION('ref_axis',(0.377700226083253,0.925927934137782,-2.49616805185365E-19));
#11720=DIRECTION('',(4.00113358033595E-18,-1.90170940755474E-18,-1.));
#11721=DIRECTION('',(-0.377700226083253,-0.925927934137781,2.49616805185365E-19));
#11722=DIRECTION('',(4.00113358033595E-18,-1.90170940755474E-18,-1.));
#11723=DIRECTION('',(0.377700226083253,0.925927934137781,-2.49616805185365E-19));
#11724=DIRECTION('center_axis',(4.00113358033595E-18,-1.90170940755474E-18,
-1.));
#11725=DIRECTION('ref_axis',(0.976179814676794,-0.216963060029996,4.31842652930035E-18));
#11726=DIRECTION('center_axis',(4.00113358033595E-18,-1.90170940755474E-18,
-1.));
#11727=DIRECTION('ref_axis',(-0.925927934137781,0.377700226083253,-4.42303742342784E-18));
#11728=DIRECTION('',(4.00113358033595E-18,-1.90170940755474E-18,-1.));
#11729=DIRECTION('center_axis',(-4.00113358033595E-18,1.90170940755474E-18,
1.));
#11730=DIRECTION('ref_axis',(-0.92592793413778,0.377700226083256,-4.42303742342784E-18));
#11731=DIRECTION('center_axis',(0.925927934137781,-0.377700226083253,4.42303742342784E-18));
#11732=DIRECTION('ref_axis',(0.377700226083253,0.925927934137781,-2.49616805185363E-19));
#11733=DIRECTION('',(-0.377700226083253,-0.925927934137781,2.49616805185364E-19));
#11734=DIRECTION('',(0.377700226083253,0.925927934137781,-2.49616805185364E-19));
#11735=DIRECTION('center_axis',(-0.925927934137781,0.377700226083253,-4.42303742342784E-18));
#11736=DIRECTION('ref_axis',(-0.377700226083253,-0.925927934137781,2.49616805185365E-19));
#11737=DIRECTION('',(4.00113358033595E-18,-1.90170940755474E-18,-1.));
#11738=DIRECTION('',(-0.377700226083253,-0.925927934137781,2.49616805185365E-19));
#11739=DIRECTION('',(0.377700226083253,0.925927934137781,-2.49616805185365E-19));
#11740=DIRECTION('center_axis',(-0.999957006340362,0.00927283510161242,
-4.01859579470807E-18));
#11741=DIRECTION('ref_axis',(-0.00927283510161242,-0.999957006340362,1.86452579419776E-18));
#11742=DIRECTION('',(0.00927283510161242,0.999957006340362,-1.86452579419776E-18));
#11743=DIRECTION('',(-4.00113358033595E-18,1.90170940755474E-18,1.));
#11744=DIRECTION('',(-0.00927283510161242,-0.999957006340362,1.86452579419776E-18));
#11745=DIRECTION('center_axis',(0.999957006340363,-0.00927283510148229,
-5.79011228582622E-14));
#11746=DIRECTION('ref_axis',(0.00927283510148229,0.999957006340363,-1.18393654034962E-11));
#11747=DIRECTION('',(0.00927283510161242,0.999957006340362,-1.86452579419776E-18));
#11748=DIRECTION('',(-0.0087838870263115,-0.947230192127013,-0.320433778574812));
#11749=DIRECTION('center_axis',(-0.129181085459131,-0.316686004743042,-0.939692620785909));
#11750=DIRECTION('ref_axis',(0.354922115319603,0.870087647088815,-0.342020143325666));
#11751=DIRECTION('',(0.925927934137781,-0.377700226083253,4.42303742342784E-18));
#11752=DIRECTION('center_axis',(-0.129181085459303,-0.316686004743113,-0.939692620785862));
#11753=DIRECTION('ref_axis',(-0.0335289983800865,0.948485905659743,-0.315040145112406));
#11754=DIRECTION('center_axis',(-0.129181085459041,-0.31668600474309,-0.939692620785906));
#11755=DIRECTION('ref_axis',(-0.251599743391323,0.927090266008532,-0.277851053259925));
#11756=DIRECTION('center_axis',(-4.00113358033595E-18,1.90170940755474E-18,
1.));
#11757=DIRECTION('ref_axis',(0.925927934137781,-0.377700226083253,4.42303742342784E-18));
#11758=DIRECTION('',(0.925927934137781,-0.377700226083253,4.42303742342784E-18));
#11759=DIRECTION('',(0.00927283510161242,0.999957006340362,-1.86452579419776E-18));
#11760=DIRECTION('center_axis',(-4.00113358033595E-18,1.90170940755474E-18,
1.));
#11761=DIRECTION('ref_axis',(0.925927934137781,-0.377700226083253,4.42303742342784E-18));
#11762=DIRECTION('',(0.204644651309627,-0.978836332943542,2.68027284920621E-18));
#11763=DIRECTION('center_axis',(-4.00113358033595E-18,1.90170940755474E-18,
1.));
#11764=DIRECTION('ref_axis',(0.925927934137781,-0.377700226083253,4.42303742342784E-18));
#11765=DIRECTION('center_axis',(4.00113358033595E-18,-1.90170940755474E-18,
-1.));
#11766=DIRECTION('ref_axis',(0.925927934137782,-0.377700226083252,4.42303742342784E-18));
#11767=DIRECTION('',(-0.00927283510161242,-0.999957006340362,1.86452579419776E-18));
#11768=DIRECTION('',(-0.204644651309627,0.978836332943542,-2.68027284920621E-18));
#11769=DIRECTION('center_axis',(-0.129181085459131,-0.316686004743042,0.939692620785909));
#11770=DIRECTION('ref_axis',(-0.354922115319603,-0.870087647088815,-0.342020143325666));
#11771=DIRECTION('center_axis',(-0.129181085458924,-0.316686004742943,0.939692620785971));
#11772=DIRECTION('ref_axis',(0.0335289983807529,-0.948485905659807,-0.315040145112141));
#11773=DIRECTION('center_axis',(-0.129181085459094,-0.316686004743076,0.939692620785903));
#11774=DIRECTION('ref_axis',(0.251599743391407,-0.927090266008522,-0.277851053259883));
#11775=DIRECTION('center_axis',(0.978836332943542,0.204644651309627,3.52728026279203E-18));
#11776=DIRECTION('ref_axis',(-0.204644651309627,0.978836332943542,-2.68027284920621E-18));
#11777=DIRECTION('',(-0.204644651309627,0.978836332943542,-2.68027284920621E-18));
#11778=DIRECTION('',(4.00113358033595E-18,-1.90170940755474E-18,-1.));
#11779=DIRECTION('',(0.204644651309627,-0.978836332943542,2.68027284920621E-18));
#11780=DIRECTION('center_axis',(0.978836332943539,0.204644651309642,-1.5115104670406E-14));
#11781=DIRECTION('ref_axis',(0.204644651309642,-0.978836332943539,-3.3090080010939E-12));
#11782=DIRECTION('center_axis',(0.978836332943534,0.204644651309665,3.08136968372797E-14));
#11783=DIRECTION('ref_axis',(0.204644651309665,-0.978836332943534,2.52482791984225E-12));
#11784=DIRECTION('center_axis',(4.00113358033595E-18,-1.90170940755474E-18,
-1.));
#11785=DIRECTION('ref_axis',(-0.925927934137781,0.377700226083253,-4.42303742342784E-18));
#11786=DIRECTION('center_axis',(-4.00113358033595E-18,1.90170940755474E-18,
1.));
#11787=DIRECTION('ref_axis',(-0.925927934137783,0.377700226083249,-4.42303742342784E-18));
#11788=DIRECTION('',(-0.377700226083253,-0.925927934137781,2.49616805185364E-19));
#11789=DIRECTION('center_axis',(4.00113358033595E-18,-1.90170940755474E-18,
-1.));
#11790=DIRECTION('ref_axis',(-0.925927934137781,0.377700226083253,-4.42303742342784E-18));
#11791=DIRECTION('',(-0.377700226083253,-0.925927934137781,2.49616805185365E-19));
#11792=DIRECTION('',(-0.925927934137781,0.377700226083253,-4.42303742342784E-18));
#11793=DIRECTION('center_axis',(4.00113358033595E-18,-1.90170940755474E-18,
-1.));
#11794=DIRECTION('ref_axis',(-0.925927934137781,0.377700226083253,-4.42303742342784E-18));
#11795=DIRECTION('center_axis',(-4.00113358033595E-18,1.90170940755474E-18,
1.));
#11796=DIRECTION('ref_axis',(-0.925927934137783,0.377700226083249,-4.42303742342784E-18));
#11797=DIRECTION('',(-0.925927934137781,0.377700226083253,-4.42303742342784E-18));
#11798=DIRECTION('',(-0.377700226083253,-0.925927934137781,2.49616805185365E-19));
#11799=DIRECTION('center_axis',(4.00113358033595E-18,-1.90170940755474E-18,
-1.));
#11800=DIRECTION('ref_axis',(-0.925927934137781,0.377700226083253,-4.42303742342784E-18));
#11801=DIRECTION('',(-0.377700226083253,-0.925927934137781,2.49616805185364E-19));
#11802=DIRECTION('center_axis',(0.925927934137782,-0.377700226083253,4.42303742342784E-18));
#11803=DIRECTION('ref_axis',(0.377700226083253,0.925927934137782,-2.49616805185365E-19));
#11804=DIRECTION('',(0.354922115319602,0.870087647088815,-0.342020143325666));
#11805=DIRECTION('',(-0.377700226083253,-0.925927934137781,2.49616805185365E-19));
#11806=DIRECTION('',(4.00113358033595E-18,-1.90170940755474E-18,-1.));
#11807=DIRECTION('',(-0.377700226083253,-0.925927934137781,2.49616805185365E-19));
#11808=DIRECTION('',(-0.354922115319602,-0.870087647088815,-0.342020143325666));
#11809=DIRECTION('',(4.00113358033595E-18,-1.90170940755474E-18,-1.));
#11810=DIRECTION('center_axis',(4.00113358033595E-18,-1.90170940755474E-18,
-1.));
#11811=DIRECTION('ref_axis',(0.975866572214553,-0.218367656108268,4.31984433794175E-18));
#11812=DIRECTION('',(4.00113358033595E-18,-1.90170940755474E-18,-1.));
#11813=DIRECTION('center_axis',(0.925927934137781,-0.377700226083253,4.42303742342784E-18));
#11814=DIRECTION('ref_axis',(0.377700226083253,0.925927934137781,-2.49616805185363E-19));
#11815=DIRECTION('center_axis',(-0.129181085459131,-0.316686004743042,-0.939692620785909));
#11816=DIRECTION('ref_axis',(0.354922115319603,0.870087647088815,-0.342020143325666));
#11817=DIRECTION('',(0.925927934137781,-0.377700226083253,4.42303742342784E-18));
#11818=DIRECTION('center_axis',(-4.00113358033595E-18,1.90170940755474E-18,
1.));
#11819=DIRECTION('ref_axis',(0.925927934137781,-0.377700226083253,4.42303742342784E-18));
#11820=DIRECTION('',(0.204644651309627,-0.978836332943542,2.68027284920621E-18));
#11821=DIRECTION('',(0.925927934137781,-0.377700226083253,4.42303742342784E-18));
#11822=DIRECTION('',(0.925927934137781,-0.377700226083253,4.42303742342784E-18));
#11823=DIRECTION('center_axis',(-4.00113358033595E-18,1.90170940755474E-18,
1.));
#11824=DIRECTION('ref_axis',(0.925927934137781,-0.377700226083253,4.42303742342784E-18));
#11825=DIRECTION('',(0.925927934137781,-0.377700226083253,4.42303742342784E-18));
#11826=DIRECTION('',(0.204644651309627,-0.978836332943542,2.68027284920621E-18));
#11827=DIRECTION('center_axis',(-0.129181085459131,-0.316686004743042,0.939692620785909));
#11828=DIRECTION('ref_axis',(-0.354922115319603,-0.870087647088815,-0.342020143325666));
#11829=DIRECTION('center_axis',(0.978836332943542,0.204644651309627,3.52728026279203E-18));
#11830=DIRECTION('ref_axis',(-0.204644651309627,0.978836332943542,-2.68027284920621E-18));
#11831=DIRECTION('',(4.00113358033595E-18,-1.90170940755474E-18,-1.));
#11832=DIRECTION('center_axis',(4.00113358033595E-18,-1.90170940755474E-18,
-1.));
#11833=DIRECTION('ref_axis',(0.976179814676794,-0.216963060029996,0.));
#11834=DIRECTION('center_axis',(0.377700226083253,0.925927934137781,-2.49616805185365E-19));
#11835=DIRECTION('ref_axis',(-0.925927934137782,0.377700226083253,-1.80221867215748E-34));
#11836=DIRECTION('center_axis',(4.00113358033595E-18,-1.90170940755474E-18,
-1.));
#11837=DIRECTION('ref_axis',(0.976179814676794,-0.216963060029996,0.));
#11838=DIRECTION('center_axis',(-0.377700226083253,-0.925927934137781,2.49616805185365E-19));
#11839=DIRECTION('ref_axis',(0.925927934137782,-0.377700226083253,4.55848320526634E-35));
#11840=DIRECTION('center_axis',(0.377700226083253,0.925927934137781,-2.49616805185364E-19));
#11841=DIRECTION('ref_axis',(-0.925927934137781,0.377700226083253,-1.53241463292932E-34));
#11842=DIRECTION('center_axis',(-0.377700226083253,-0.925927934137781,2.49616805185364E-19));
#11843=DIRECTION('ref_axis',(0.925927934137781,-0.377700226083253,1.53241463292932E-34));
#11844=DIRECTION('center_axis',(0.204644651309627,-0.978836332943542,2.68027284920621E-18));
#11845=DIRECTION('ref_axis',(0.978836332943542,0.204644651309627,-3.8498424257767E-34));
#11846=DIRECTION('',(0.204644651309627,-0.978836332943542,2.68027284920621E-18));
#11847=DIRECTION('center_axis',(-0.204644651309626,0.978836332943543,-2.68027284920621E-18));
#11848=DIRECTION('ref_axis',(-0.978836332943543,-0.204644651309626,2.50909234811124E-33));
#11849=DIRECTION('center_axis',(-0.377700226083253,-0.925927934137781,2.49616805185365E-19));
#11850=DIRECTION('ref_axis',(0.925927934137781,-0.377700226083253,-3.31576666279908E-34));
#11851=DIRECTION('center_axis',(-4.00113358033595E-18,1.90170940755474E-18,
1.));
#11852=DIRECTION('ref_axis',(-0.0982550627361708,0.99516126464343,0.));
#11853=DIRECTION('center_axis',(-4.00113358033595E-18,1.90170940755474E-18,
1.));
#11854=DIRECTION('ref_axis',(0.925927934137781,-0.377700226083253,4.42303742342784E-18));
#11855=DIRECTION('center_axis',(-0.00927283510160954,-0.999957006340362,
1.86452579419778E-18));
#11856=DIRECTION('ref_axis',(0.999957006340362,-0.00927283510160953,2.50052584644563E-34));
#11857=DIRECTION('center_axis',(0.00927283510161242,0.999957006340362,-1.86452579419776E-18));
#11858=DIRECTION('ref_axis',(-0.999957006340362,0.00927283510161242,-2.38242583230871E-34));
#11859=DIRECTION('',(0.00927283510161242,0.999957006340362,-1.86452579419776E-18));
#11860=DIRECTION('center_axis',(-0.204644651309627,0.978836332943542,-2.68027284920621E-18));
#11861=DIRECTION('ref_axis',(-0.978836332943542,-0.204644651309627,3.8498424257767E-34));
#11862=DIRECTION('center_axis',(-0.204644651309626,0.978836332943543,-2.68027284920621E-18));
#11863=DIRECTION('ref_axis',(-0.978836332943543,-0.204644651309626,2.50909234811124E-33));
#11864=DIRECTION('',(-0.204644651309627,0.978836332943542,-2.68027284920621E-18));
#11865=DIRECTION('center_axis',(0.377700226083253,0.925927934137781,-2.49616805185365E-19));
#11866=DIRECTION('ref_axis',(-0.925927934137781,0.377700226083253,3.31576666279908E-34));
#11867=DIRECTION('center_axis',(-4.00113358033595E-18,1.90170940755474E-18,
1.));
#11868=DIRECTION('ref_axis',(-0.0982550627361708,0.99516126464343,0.));
#11869=DIRECTION('center_axis',(-0.0092728351016097,-0.999957006340362,
-2.115631353514E-16));
#11870=DIRECTION('ref_axis',(0.999957006340362,-0.0092728351016097,-6.33219768041088E-32));
#11871=DIRECTION('center_axis',(4.00113358033595E-18,-1.90170940755474E-18,
-1.));
#11872=DIRECTION('ref_axis',(0.925927934137781,-0.377700226083253,4.42303742342784E-18));
#11873=DIRECTION('center_axis',(-0.00927283510161242,-0.999957006340362,
1.86452579419776E-18));
#11874=DIRECTION('ref_axis',(0.999957006340362,-0.00927283510161242,-8.42037297766392E-34));
#11875=DIRECTION('',(-0.00927283510161242,-0.999957006340362,1.86452579419776E-18));
#11876=DIRECTION('center_axis',(4.00113358033595E-18,-1.90170940755474E-18,
-1.));
#11877=DIRECTION('ref_axis',(-0.925927934137781,0.377700226083255,-4.42303742342784E-18));
#11878=DIRECTION('center_axis',(-0.377700226083253,-0.925927934137781,2.49616805185364E-19));
#11879=DIRECTION('ref_axis',(4.00113358033594E-18,-1.90170940755474E-18,
-1.));
#11880=DIRECTION('',(0.925927934137781,-0.377700226083253,4.42303742342784E-18));
#11881=DIRECTION('',(0.925927934137781,-0.377700226083253,4.42303742342784E-18));
#11882=DIRECTION('center_axis',(5.31244646680575E-17,1.18523594394076E-16,
-1.));
#11883=DIRECTION('ref_axis',(0.377700226083253,0.925927934137781,1.29809429219568E-16));
#11884=DIRECTION('center_axis',(-8.58733520598719E-17,-1.98807130261829E-16,
1.));
#11885=DIRECTION('ref_axis',(-0.377700226083253,-0.925927934137781,-2.16515459902737E-16));
#45245=CARTESIAN_POINT('',(0.,0.,0.));
#45246=CARTESIAN_POINT('Origin',(-31.229031910667,-116.780702189177,178.985485069079));
#45247=CARTESIAN_POINT('',(-81.9809794708757,-61.5607798889249,178.985485069079));
#45248=CARTESIAN_POINT('',(-104.027257502361,-98.7413465825904,178.985485069079));
#45249=CARTESIAN_POINT('Origin',(-31.229031910667,-116.780702189177,178.985485069079));
#45250=CARTESIAN_POINT('',(-83.2437717586763,-60.6850977397733,180.485485069079));
#45251=CARTESIAN_POINT('Ctrl Pts',(-83.2437717586763,-60.6850977397733,
180.485485069079));
#45252=CARTESIAN_POINT('Ctrl Pts',(-83.2422325967899,-60.6861625729165,
180.485485069079));
#45253=CARTESIAN_POINT('Ctrl Pts',(-83.2406934401744,-60.6872274114438,
180.485481729905));
#45254=CARTESIAN_POINT('Ctrl Pts',(-83.070898721105,-60.8046979074495,180.484744993636));
#45255=CARTESIAN_POINT('Ctrl Pts',(-82.9042059840165,-60.9201343030104,
180.444117117279));
#45256=CARTESIAN_POINT('Ctrl Pts',(-82.5956424548927,-61.1339972589321,
180.288086830727));
#45257=CARTESIAN_POINT('Ctrl Pts',(-82.4561538201594,-61.2307685378217,
180.174971263388));
#45258=CARTESIAN_POINT('Ctrl Pts',(-82.2247684030825,-61.3913855449473,
179.892696719416));
#45259=CARTESIAN_POINT('Ctrl Pts',(-82.1339882775335,-61.4544507205017,
179.72770850648));
#45260=CARTESIAN_POINT('Ctrl Pts',(-82.0121144592395,-61.5391347772565,
179.368058467365));
#45261=CARTESIAN_POINT('Ctrl Pts',(-81.9809990073737,-61.5607663092965,
179.17792947018));
#45262=CARTESIAN_POINT('Ctrl Pts',(-81.9809794739406,-61.5607798867945,
178.985605775658));
#45263=CARTESIAN_POINT('Ctrl Pts',(-81.9809794708757,-61.5607798889249,
178.985545422265));
#45264=CARTESIAN_POINT('Ctrl Pts',(-81.9809794708757,-61.5607798889249,
178.985485069079));
#45265=CARTESIAN_POINT('',(-106.601824441649,-103.696660532197,180.485485069079));
#45266=CARTESIAN_POINT('Origin',(-31.229031910667,-116.780702189177,180.485485069079));
#45267=CARTESIAN_POINT('',(-105.613710699518,-102.630519079741,180.265888107377));
#45268=CARTESIAN_POINT('Ctrl Pts',(-105.613710699518,-102.630519079741,
180.265888107377));
#45269=CARTESIAN_POINT('Ctrl Pts',(-105.658052765278,-102.739223164379,
180.280074653183));
#45270=CARTESIAN_POINT('Ctrl Pts',(-105.708972522035,-102.837432096684,
180.298606216492));
#45271=CARTESIAN_POINT('Ctrl Pts',(-105.889297996009,-103.133428559691,
180.362418620409));
#45272=CARTESIAN_POINT('Ctrl Pts',(-106.053691035723,-103.31971416131,180.41853554034));
#45273=CARTESIAN_POINT('Ctrl Pts',(-106.358503600507,-103.559189420194,
180.472850239938));
#45274=CARTESIAN_POINT('Ctrl Pts',(-106.47665098808,-103.634137304981,180.485485069079));
#45275=CARTESIAN_POINT('Ctrl Pts',(-106.601824441649,-103.696660532197,
180.485485069079));
#45276=CARTESIAN_POINT('Ctrl Pts',(-104.027257502361,-98.7413465825906,
178.985485069079));
#45277=CARTESIAN_POINT('Ctrl Pts',(-104.027257502361,-98.7413465825906,
179.026424101808));
#45278=CARTESIAN_POINT('Ctrl Pts',(-104.032888367115,-98.7551505853665,
179.073234241807));
#45279=CARTESIAN_POINT('Ctrl Pts',(-104.053185991761,-98.8049099880857,
179.167298560279));
#45280=CARTESIAN_POINT('Ctrl Pts',(-104.075243416314,-98.858983520846,179.223244697426));
#45281=CARTESIAN_POINT('Ctrl Pts',(-104.152999108407,-99.0496007415273,
179.382318294648));
#45282=CARTESIAN_POINT('Ctrl Pts',(-104.224794456088,-99.2256062436916,
179.466142077644));
#45283=CARTESIAN_POINT('Ctrl Pts',(-104.37241425056,-99.5874945400008,179.616310592306));
#45284=CARTESIAN_POINT('Ctrl Pts',(-104.448792282881,-99.7747344429623,
179.678812502117));
#45285=CARTESIAN_POINT('Ctrl Pts',(-104.856768027367,-100.774882476199,
179.982161235303));
#45286=CARTESIAN_POINT('Ctrl Pts',(-105.232613956139,-101.696264620951,
180.143962204427));
#45287=CARTESIAN_POINT('Ctrl Pts',(-105.613710699518,-102.630519079741,
180.265888107377));
#45288=CARTESIAN_POINT('Origin',(-31.229031910667,-116.780702189177,172.985485069079));
#45289=CARTESIAN_POINT('',(-83.2437717586763,-60.6850977397733,171.485485069079));
#45290=CARTESIAN_POINT('',(-106.601824441649,-103.696660532197,171.485485069079));
#45291=CARTESIAN_POINT('Origin',(-31.229031910667,-116.780702189177,171.485485069079));
#45292=CARTESIAN_POINT('',(-81.9809794708757,-61.5607798889249,172.985485069079));
#45293=CARTESIAN_POINT('Ctrl Pts',(-81.9809794708757,-61.5607798889249,
172.985485069079));
#45294=CARTESIAN_POINT('Ctrl Pts',(-81.9809794708757,-61.5607798889249,
172.794647159443));
#45295=CARTESIAN_POINT('Ctrl Pts',(-82.0116164204235,-61.5394810565551,
172.605891278582));
#45296=CARTESIAN_POINT('Ctrl Pts',(-82.1311013468671,-61.4564564904976,
172.250286109186));
#45297=CARTESIAN_POINT('Ctrl Pts',(-82.2194216547433,-61.3950995397068,
172.08752918528));
#45298=CARTESIAN_POINT('Ctrl Pts',(-82.4445214808283,-61.2388407613391,
171.807588409535));
#45299=CARTESIAN_POINT('Ctrl Pts',(-82.5802654678823,-61.1446627802494,
171.694380155136));
#45300=CARTESIAN_POINT('Ctrl Pts',(-82.809839687611,-60.9855353654994,171.572921494192));
#45301=CARTESIAN_POINT('Ctrl Pts',(-82.8932820097023,-60.927723055843,171.540639437838));
#45302=CARTESIAN_POINT('Ctrl Pts',(-83.0643730653962,-60.8092421044008,
171.497047848165));
#45303=CARTESIAN_POINT('Ctrl Pts',(-83.1516444302605,-60.7488349303393,
171.485874790325));
#45304=CARTESIAN_POINT('Ctrl Pts',(-83.2406934401744,-60.6872274114439,
171.485488408253));
#45305=CARTESIAN_POINT('Ctrl Pts',(-83.2422325967899,-60.6861625729165,
171.485485069079));
#45306=CARTESIAN_POINT('Ctrl Pts',(-83.2437717586764,-60.6850977397733,
171.485485069079));
#45307=CARTESIAN_POINT('',(-104.027257502361,-98.7413465825904,172.985485069079));
#45308=CARTESIAN_POINT('Origin',(-31.229031910667,-116.780702189177,172.985485069079));
#45309=CARTESIAN_POINT('',(-105.613710699519,-102.630519079742,171.705082030781));
#45310=CARTESIAN_POINT('Ctrl Pts',(-105.613710699519,-102.630519079742,
171.705082030781));
#45311=CARTESIAN_POINT('Ctrl Pts',(-105.232613956139,-101.696264620952,
171.827007933732));
#45312=CARTESIAN_POINT('Ctrl Pts',(-104.856768027367,-100.7748824762,171.988808902855));
#45313=CARTESIAN_POINT('Ctrl Pts',(-104.448792282881,-99.7747344429622,
172.292157636041));
#45314=CARTESIAN_POINT('Ctrl Pts',(-104.37241425056,-99.5874945400007,172.354659545853));
#45315=CARTESIAN_POINT('Ctrl Pts',(-104.224794456088,-99.2256062436915,
172.504828060515));
#45316=CARTESIAN_POINT('Ctrl Pts',(-104.152999108407,-99.0496007415272,
172.58865184351));
#45317=CARTESIAN_POINT('Ctrl Pts',(-104.075243416314,-98.8589835208459,
172.747725440733));
#45318=CARTESIAN_POINT('Ctrl Pts',(-104.053185991761,-98.8049099880857,
172.803671577879));
#45319=CARTESIAN_POINT('Ctrl Pts',(-104.032888367115,-98.7551505853665,
172.897735896352));
#45320=CARTESIAN_POINT('Ctrl Pts',(-104.027257502361,-98.7413465825906,
172.94454603635));
#45321=CARTESIAN_POINT('Ctrl Pts',(-104.027257502361,-98.7413465825906,
172.985485069079));
#45322=CARTESIAN_POINT('Ctrl Pts',(-106.601824441649,-103.696660532197,
171.485485069079));
#45323=CARTESIAN_POINT('Ctrl Pts',(-106.53220525908,-103.66188625821,171.485485069079));
#45324=CARTESIAN_POINT('Ctrl Pts',(-106.464169344039,-103.622977573215,
171.489410638421));
#45325=CARTESIAN_POINT('Ctrl Pts',(-106.211695162338,-103.458610972797,
171.516115265147));
#45326=CARTESIAN_POINT('Ctrl Pts',(-106.046375023087,-103.308026666015,
171.559682835566));
#45327=CARTESIAN_POINT('Ctrl Pts',(-105.804368479235,-103.003327965471,
171.637167539166));
#45328=CARTESIAN_POINT('Ctrl Pts',(-105.715452773286,-102.858679667203,
171.670867024465));
#45329=CARTESIAN_POINT('Ctrl Pts',(-105.634000122074,-102.67893082039,171.698474541123));
#45330=CARTESIAN_POINT('Ctrl Pts',(-105.623629484128,-102.654834870701,
171.701908671809));
#45331=CARTESIAN_POINT('Ctrl Pts',(-105.613710699519,-102.630519079742,
171.705082030781));
#45332=CARTESIAN_POINT('Origin',(106.899307254449,-150.793932399799,177.485485069079));
#45333=CARTESIAN_POINT('',(-91.410849784583,-57.8787323612094,180.485485069079));
#45334=CARTESIAN_POINT('',(-107.009977058815,-103.84909152684,180.485485069079));
#45335=CARTESIAN_POINT('Origin',(106.899307254449,-150.793932399799,180.485485069079));
#45336=CARTESIAN_POINT('',(-94.1292986217245,-56.6052939157322,177.485485069079));
#45337=CARTESIAN_POINT('Ctrl Pts',(-94.1292986217245,-56.6052939157322,
177.485485069079));
#45338=CARTESIAN_POINT('Ctrl Pts',(-94.1292986217245,-56.6052939157322,
177.856763201439));
#45339=CARTESIAN_POINT('Ctrl Pts',(-94.0660385633859,-56.6351180251081,
178.239317280815));
#45340=CARTESIAN_POINT('Ctrl Pts',(-93.8670456578475,-56.7283483675185,
178.785738776833));
#45341=CARTESIAN_POINT('Ctrl Pts',(-93.7835242707107,-56.7674422240991,
178.963188566011));
#45342=CARTESIAN_POINT('Ctrl Pts',(-93.6330340156095,-56.8378730704672,
179.215996936763));
#45343=CARTESIAN_POINT('Ctrl Pts',(-93.5786828002802,-56.8633094959559,
179.298034924651));
#45344=CARTESIAN_POINT('Ctrl Pts',(-93.491075623674,-56.9043212188128,179.416933247598));
#45345=CARTESIAN_POINT('Ctrl Pts',(-93.4457533491126,-56.9255407794407,
179.475342645356));
#45346=CARTESIAN_POINT('Ctrl Pts',(-93.3902788233905,-56.9515217739284,
179.541489655834));
#45347=CARTESIAN_POINT('Ctrl Pts',(-93.3619004743536,-56.96481499421,179.574041689426));
#45348=CARTESIAN_POINT('Ctrl Pts',(-93.3475521299737,-56.9715368357171,
179.590184575139));
#45349=CARTESIAN_POINT('Ctrl Pts',(-93.3413688531149,-56.9744336964136,
179.597074130901));
#45350=CARTESIAN_POINT('Ctrl Pts',(-93.3372391296956,-56.9763685027338,
179.601660729943));
#45351=CARTESIAN_POINT('Ctrl Pts',(-93.3344333984817,-56.977683037912,179.604764185584));
#45352=CARTESIAN_POINT('Ctrl Pts',(-93.1621805239265,-57.0583876466175,
179.794841788008));
#45353=CARTESIAN_POINT('Ctrl Pts',(-92.9270395815964,-57.1691883844647,
180.005835194439));
#45354=CARTESIAN_POINT('Ctrl Pts',(-92.4482315155942,-57.3936123286524,
180.265019693198));
#45355=CARTESIAN_POINT('Ctrl Pts',(-92.2678586301383,-57.4780238050178,
180.341232854623));
#45356=CARTESIAN_POINT('Ctrl Pts',(-91.8674994509229,-57.6652677007972,
180.451346123991));
#45357=CARTESIAN_POINT('Ctrl Pts',(-91.6474047383563,-57.7681443459078,
180.485147996224));
#45358=CARTESIAN_POINT('Ctrl Pts',(-91.4113312145148,-57.878670006244,180.485485069079));
#45359=CARTESIAN_POINT('',(-109.534287722621,-101.392525888427,177.485485069079));
#45360=CARTESIAN_POINT('Origin',(106.899307254449,-150.793932399799,177.485485069079));
#45361=CARTESIAN_POINT('Ctrl Pts',(-107.009977058815,-103.84909152684,180.485485069079));
#45362=CARTESIAN_POINT('Ctrl Pts',(-107.137921837196,-103.881980428467,
180.485485069079));
#45363=CARTESIAN_POINT('Ctrl Pts',(-107.268759891508,-103.902517901244,
180.478513657667));
#45364=CARTESIAN_POINT('Ctrl Pts',(-107.618867465629,-103.923371702875,
180.436712848229));
#45365=CARTESIAN_POINT('Ctrl Pts',(-107.831376286747,-103.901466369003,
180.387630831655));
#45366=CARTESIAN_POINT('Ctrl Pts',(-108.256149207338,-103.793261446598,
180.232967049603));
#45367=CARTESIAN_POINT('Ctrl Pts',(-108.457219871836,-103.702395545817,
180.124910466337));
#45368=CARTESIAN_POINT('Ctrl Pts',(-108.86130608821,-103.444418866416,179.830873029469));
#45369=CARTESIAN_POINT('Ctrl Pts',(-109.044027201329,-103.26519727749,179.634119786442));
#45370=CARTESIAN_POINT('Ctrl Pts',(-109.370932552757,-102.820739354799,
179.1432271976));
#45371=CARTESIAN_POINT('Ctrl Pts',(-109.48673079434,-102.54337787575,178.835080933563));
#45372=CARTESIAN_POINT('Ctrl Pts',(-109.603841517271,-101.97541853432,178.18613896477));
#45373=CARTESIAN_POINT('Ctrl Pts',(-109.598798782044,-101.679242827835,
177.838268930735));
#45374=CARTESIAN_POINT('Ctrl Pts',(-109.535241658531,-101.396720316011,
177.490648716974));
#45375=CARTESIAN_POINT('Ctrl Pts',(-109.534766330367,-101.39462272741,177.488066892411));
#45376=CARTESIAN_POINT('Ctrl Pts',(-109.534287722621,-101.392525888427,
177.485485069079));
#45377=CARTESIAN_POINT('Origin',(106.899307254449,-150.793932399799,174.485485069079));
#45378=CARTESIAN_POINT('',(-94.1292986217245,-56.6052939157322,174.485485069079));
#45379=CARTESIAN_POINT('',(-109.534287722621,-101.392525888427,174.485485069079));
#45380=CARTESIAN_POINT('Origin',(106.899307254449,-150.793932399799,174.485485069079));
#45381=CARTESIAN_POINT('',(-91.4108060345764,-57.8786324516506,171.485485069079));
#45382=CARTESIAN_POINT('Ctrl Pts',(-91.410862632993,-57.8787562475091,171.485488161254));
#45383=CARTESIAN_POINT('Ctrl Pts',(-91.6484623587964,-57.7676500200356,
171.485988398864));
#45384=CARTESIAN_POINT('Ctrl Pts',(-91.8679492309091,-57.6650573954028,
171.519752422514));
#45385=CARTESIAN_POINT('Ctrl Pts',(-92.2677947733545,-57.4780539094026,
171.629714980247));
#45386=CARTESIAN_POINT('Ctrl Pts',(-92.4481639960319,-57.3936442958883,
171.705919699708));
#45387=CARTESIAN_POINT('Ctrl Pts',(-92.7673736667778,-57.2440265817481,
171.878699917269));
#45388=CARTESIAN_POINT('Ctrl Pts',(-92.9063177114656,-57.1787762224701,
171.975241718896));
#45389=CARTESIAN_POINT('Ctrl Pts',(-93.0863798448037,-57.0941626545074,
172.122130842798));
#45390=CARTESIAN_POINT('Ctrl Pts',(-93.1417074499794,-57.0681551828317,
172.171477751684));
#45391=CARTESIAN_POINT('Ctrl Pts',(-93.2181992503479,-57.03221925648,172.244767934548));
#45392=CARTESIAN_POINT('Ctrl Pts',(-93.2548217785949,-57.0150194895201,
172.281233967651));
#45393=CARTESIAN_POINT('Ctrl Pts',(-93.2948376449404,-56.9962442115694,
172.323214494815));
#45394=CARTESIAN_POINT('Ctrl Pts',(-93.3141848810401,-56.9871724551456,
172.344035313164));
#45395=CARTESIAN_POINT('Ctrl Pts',(-93.3236954404761,-56.9827146845638,
172.354399845872));
#45396=CARTESIAN_POINT('Ctrl Pts',(-93.3277366813326,-56.9808208558246,
172.358831588447));
#45397=CARTESIAN_POINT('Ctrl Pts',(-93.3304231532481,-56.9795619917248,
172.361783776208));
#45398=CARTESIAN_POINT('Ctrl Pts',(-93.3310258878557,-56.9792795491844,
172.362445828695));
#45399=CARTESIAN_POINT('Ctrl Pts',(-93.5983418840511,-56.8540342037519,
172.657424206742));
#45400=CARTESIAN_POINT('Ctrl Pts',(-93.8006909816924,-56.7594348190334,
173.003045307483));
#45401=CARTESIAN_POINT('Ctrl Pts',(-94.0660265072745,-56.6351229429811,
173.731602247926));
#45402=CARTESIAN_POINT('Ctrl Pts',(-94.1292986217245,-56.6052939157322,
174.114172392865));
#45403=CARTESIAN_POINT('Ctrl Pts',(-94.1292986217245,-56.6052939157322,
174.485485069079));
#45404=CARTESIAN_POINT('',(-107.009977058815,-103.84909152684,171.485485069079));
#45405=CARTESIAN_POINT('Origin',(106.899307254449,-150.793932399799,171.485485069079));
#45406=CARTESIAN_POINT('Ctrl Pts',(-109.534287722621,-101.392525888427,
174.485485069079));
#45407=CARTESIAN_POINT('Ctrl Pts',(-109.534766330367,-101.39462272741,174.482903245747));
#45408=CARTESIAN_POINT('Ctrl Pts',(-109.535241658531,-101.396720316011,
174.480321421184));
#45409=CARTESIAN_POINT('Ctrl Pts',(-109.598798782043,-101.679242827829,
174.132701207431));
#45410=CARTESIAN_POINT('Ctrl Pts',(-109.60384151727,-101.975418534307,173.784831173405));
#45411=CARTESIAN_POINT('Ctrl Pts',(-109.486730794348,-102.543377875726,
173.135889204623));
#45412=CARTESIAN_POINT('Ctrl Pts',(-109.370932552772,-102.820739354769,
172.827742940592));
#45413=CARTESIAN_POINT('Ctrl Pts',(-109.044027201355,-103.265197277462,
172.336850351747));
#45414=CARTESIAN_POINT('Ctrl Pts',(-108.861306088238,-103.444418866393,
172.140097108715));
#45415=CARTESIAN_POINT('Ctrl Pts',(-108.457219871866,-103.702395545801,
171.846059671839));
#45416=CARTESIAN_POINT('Ctrl Pts',(-108.256149207368,-103.793261446586,
171.73800308857));
#45417=CARTESIAN_POINT('Ctrl Pts',(-107.831376286778,-103.901466368998,
171.583339306512));
#45418=CARTESIAN_POINT('Ctrl Pts',(-107.618867465661,-103.923371702873,
171.534257289936));
#45419=CARTESIAN_POINT('Ctrl Pts',(-107.268759891529,-103.902517901247,
171.492456480493));
#45420=CARTESIAN_POINT('Ctrl Pts',(-107.137921837206,-103.88198042847,171.485485069079));
#45421=CARTESIAN_POINT('Ctrl Pts',(-107.009977058815,-103.84909152684,171.485485069079));
#45422=CARTESIAN_POINT('Origin',(106.899307254449,-150.793932399799,180.485485069079));
#45423=CARTESIAN_POINT('',(-92.5715804833908,-57.2874890652447,178.785485069079));
#45424=CARTESIAN_POINT('',(-108.319971216218,-103.75403258522,178.785485069079));
#45425=CARTESIAN_POINT('Origin',(106.899307254449,-150.793932399799,178.785485069079));
#45426=CARTESIAN_POINT('',(-108.319971216218,-103.75403258522,173.185485069079));
#45427=CARTESIAN_POINT('',(-108.319971216218,-103.75403258522,180.485485069079));
#45428=CARTESIAN_POINT('',(-92.5715804833908,-57.2874890652447,173.185485069079));
#45429=CARTESIAN_POINT('Origin',(106.899307254449,-150.793932399799,173.185485069079));
#45430=CARTESIAN_POINT('',(-92.5715804833908,-57.2874890652447,178.785485069079));
#45431=CARTESIAN_POINT('Origin',(-70.143810135276,-11.0431453779933,170.985485069079));
#45432=CARTESIAN_POINT('',(-71.9956660035516,-10.2877449258268,178.785485069079));
#45433=CARTESIAN_POINT('Origin',(-70.143810135276,-11.0431453779933,178.785485069079));
#45434=CARTESIAN_POINT('',(-71.9956660035516,-10.2877449258268,180.485485069079));
#45435=CARTESIAN_POINT('',(-71.9956660035516,-10.2877449258268,170.985485069079));
#45436=CARTESIAN_POINT('Origin',(-70.143810135276,-11.0431453779933,180.485485069079));
#45437=CARTESIAN_POINT('Origin',(-69.9391102914966,14.1820463536532,180.985485069079));
#45438=CARTESIAN_POINT('',(-68.087254423221,13.4266459014867,180.985485069079));
#45439=CARTESIAN_POINT('Origin',(-69.9391102914966,14.1820463536532,180.985485069079));
#45440=CARTESIAN_POINT('',(-68.087254423221,13.4266459014867,179.485485069079));
#45441=CARTESIAN_POINT('',(-68.087254423221,13.4266459014867,180.985485069079));
#45442=CARTESIAN_POINT('Origin',(-69.9391102914966,14.1820463536532,179.485485069079));
#45443=CARTESIAN_POINT('Origin',(-84.8548278771908,-59.0746191263193,180.485485069079));
#45444=CARTESIAN_POINT('',(-83.9288999430531,-59.4523193524025,180.485485069079));
#45445=CARTESIAN_POINT('Origin',(-84.8548278771908,-59.0746191263193,180.485485069079));
#45446=CARTESIAN_POINT('',(-83.9288999430531,-59.4523193524025,178.785485069079));
#45447=CARTESIAN_POINT('',(-83.9288999430531,-59.4523193524025,180.485485069079));
#45448=CARTESIAN_POINT('Origin',(-84.8548278771908,-59.0746191263193,178.785485069079));
#45449=CARTESIAN_POINT('Origin',(-31.229031910667,-116.780702189177,180.485485069079));
#45450=CARTESIAN_POINT('',(-104.027257502361,-98.7413465825904,178.785485069079));
#45451=CARTESIAN_POINT('',(-104.027257502361,-98.7413465825904,180.485485069079));
#45452=CARTESIAN_POINT('',(-81.9809794708757,-61.5607798889249,178.785485069079));
#45453=CARTESIAN_POINT('Origin',(-31.229031910667,-116.780702189177,178.785485069079));
#45454=CARTESIAN_POINT('',(-81.9809794708757,-61.5607798889249,180.485485069079));
#45455=CARTESIAN_POINT('Origin',(-70.143810135276,-11.0431453779933,170.985485069079));
#45456=CARTESIAN_POINT('',(-71.9956660035516,-10.2877449258268,171.485485069079));
#45457=CARTESIAN_POINT('Origin',(-70.143810135276,-11.0431453779933,171.485485069079));
#45458=CARTESIAN_POINT('',(-71.9956660035516,-10.2877449258268,173.185485069079));
#45459=CARTESIAN_POINT('',(-71.9956660035516,-10.2877449258268,170.985485069079));
#45460=CARTESIAN_POINT('Origin',(-70.143810135276,-11.0431453779933,173.185485069079));
#45461=CARTESIAN_POINT('Origin',(-69.9391102914966,14.1820463536532,180.985485069079));
#45462=CARTESIAN_POINT('',(-68.087254423221,13.4266459014867,172.485485069079));
#45463=CARTESIAN_POINT('Origin',(-69.9391102914966,14.1820463536532,172.485485069079));
#45464=CARTESIAN_POINT('',(-68.087254423221,13.4266459014867,170.985485069079));
#45465=CARTESIAN_POINT('',(-68.087254423221,13.4266459014867,180.985485069079));
#45466=CARTESIAN_POINT('Origin',(-69.9391102914966,14.1820463536532,170.985485069079));
#45467=CARTESIAN_POINT('Origin',(-84.8548278771908,-59.0746191263193,180.485485069079));
#45468=CARTESIAN_POINT('',(-83.9288999430531,-59.4523193524025,173.185485069079));
#45469=CARTESIAN_POINT('Origin',(-84.8548278771908,-59.0746191263193,173.185485069079));
#45470=CARTESIAN_POINT('',(-83.9288999430531,-59.4523193524025,171.485485069079));
#45471=CARTESIAN_POINT('',(-83.9288999430531,-59.4523193524025,180.485485069079));
#45472=CARTESIAN_POINT('Origin',(-84.8548278771908,-59.0746191263193,171.485485069079));
#45473=CARTESIAN_POINT('Origin',(-31.229031910667,-116.780702189177,180.485485069079));
#45474=CARTESIAN_POINT('',(-104.027257502361,-98.7413465825904,173.185485069079));
#45475=CARTESIAN_POINT('',(-81.9809794708757,-61.5607798889249,173.185485069079));
#45476=CARTESIAN_POINT('Origin',(-31.229031910667,-116.780702189177,173.185485069079));
#45477=CARTESIAN_POINT('',(-104.027257502361,-98.7413465825904,180.485485069079));
#45478=CARTESIAN_POINT('',(-81.9809794708757,-61.5607798889249,180.485485069079));
#45479=CARTESIAN_POINT('Origin',(106.899307254449,-150.793932399799,180.485485069079));
#45480=CARTESIAN_POINT('',(-94.1292986217245,-56.6052939157322,180.485485069079));
#45481=CARTESIAN_POINT('',(-109.534287722621,-101.392525888427,361.145530749938));
#45482=CARTESIAN_POINT('Origin',(-107.048859311027,-106.148770055693,180.485485069079));
#45483=CARTESIAN_POINT('',(-105.613710699519,-102.630519079742,173.185485069079));
#45484=CARTESIAN_POINT('',(-105.613710699519,-102.630519079742,361.145530749938));
#45485=CARTESIAN_POINT('',(-79.4940096800365,-38.5983604123683,173.185485069079));
#45486=CARTESIAN_POINT('Origin',(-107.048859311027,-106.148770055693,180.485485069079));
#45487=CARTESIAN_POINT('',(-105.613710699519,-102.630519079742,178.785485069079));
#45488=CARTESIAN_POINT('',(-105.613710699519,-102.630519079742,361.145530749938));
#45489=CARTESIAN_POINT('',(-79.4940096800365,-38.5983604123683,178.785485069079));
#45490=CARTESIAN_POINT('Origin',(-64.3046088901795,-18.2273525712768,180.485485069079));
#45491=CARTESIAN_POINT('',(-64.3046088901795,-18.2273525712768,172.985485069079));
#45492=CARTESIAN_POINT('',(-64.3046088901795,-18.2273525712768,172.985485069079));
#45493=CARTESIAN_POINT('',(-64.3046088901795,-18.2273525712768,173.185485069079));
#45494=CARTESIAN_POINT('',(-64.3046088901795,-18.2273525712768,180.485485069079));
#45495=CARTESIAN_POINT('',(-73.5957040846178,-41.004369859499,173.185485069079));
#45496=CARTESIAN_POINT('Origin',(-64.100606517944,3.77170156821119,180.485485069079));
#45497=CARTESIAN_POINT('',(-64.3024536808101,-17.9949407268459,172.485485069079));
#45498=CARTESIAN_POINT('',(-64.067029466095,7.39255839147599,172.485485069079));
#45499=CARTESIAN_POINT('',(-64.100606517944,3.77170156821119,172.485485069079));
#45500=CARTESIAN_POINT('',(-64.067029466095,7.39255839147599,172.685485069079));
#45501=CARTESIAN_POINT('',(-64.067029466095,7.39255839147599,180.485485069079));
#45502=CARTESIAN_POINT('',(-64.0976157548621,4.09421722445422,172.685485069079));
#45503=CARTESIAN_POINT('',(-64.100606517944,3.77170156821119,172.685485069079));
#45504=CARTESIAN_POINT('',(-64.1113219987316,2.61617362315227,173.185485069079));
#45505=CARTESIAN_POINT('',(-64.1222537350124,1.437325281122,173.584271796681));
#45506=CARTESIAN_POINT('',(-64.1303313887531,0.566253342026285,173.185485069079));
#45507=CARTESIAN_POINT('Origin',(-64.2669244479369,-14.1635660768473,172.985485069062));
#45508=CARTESIAN_POINT('Origin',(-178.096445811705,1.62308776542128,180.485485069079));
#45509=CARTESIAN_POINT('Origin',(-107.523469003812,-101.851499334574,180.485485069079));
#45510=CARTESIAN_POINT('',(-64.6577925771904,-15.1217749800781,180.485485069079));
#45511=CARTESIAN_POINT('',(-74.9845959858244,-40.4378195203742,180.485485069079));
#45512=CARTESIAN_POINT('',(-64.4948557181401,2.4488872837273,180.485485069079));
#45513=CARTESIAN_POINT('',(-64.6954770194348,-19.1855614746571,180.485485069079));
#45514=CARTESIAN_POINT('',(-73.9667318408259,6.31261103702609,180.485485069079));
#45515=CARTESIAN_POINT('',(-76.6565310829785,7.40982146175055,180.485485069079));
#45516=CARTESIAN_POINT('',(-73.9319567695917,6.14627830862634,180.485485069079));
#45517=CARTESIAN_POINT('',(-73.9667318408259,6.31261103702609,180.485485069079));
#45518=CARTESIAN_POINT('',(-75.1094485830761,3.25967012829823,180.485485069079));
#45519=CARTESIAN_POINT('',(-90.3736629061554,-34.16038275589,180.485485069079));
#45520=CARTESIAN_POINT('',(-85.7265587833611,-43.9488769757557,180.485485069079));
#45521=CARTESIAN_POINT('Origin',(-178.096445811705,1.62308776542128,180.485485069079));
#45522=CARTESIAN_POINT('',(-82.9662394330532,-37.1819845645561,180.485485069079));
#45523=CARTESIAN_POINT('Origin',(-178.096445811705,1.62308776542128,171.485485069079));
#45524=CARTESIAN_POINT('Origin',(-107.523469003812,-101.851499334574,171.485485069079));
#45525=CARTESIAN_POINT('',(-85.7265587833611,-43.9488769757557,171.485485069079));
#45526=CARTESIAN_POINT('',(-92.9256857780509,-61.5974573192564,171.485485069079));
#45527=CARTESIAN_POINT('',(-75.1094485830761,3.25967012829824,171.485485069079));
#45528=CARTESIAN_POINT('Origin',(-178.096445811705,1.62308776542128,171.485485069079));
#45529=CARTESIAN_POINT('',(-73.9319567695917,6.14627830862634,171.485485069079));
#45530=CARTESIAN_POINT('',(-73.3598858593218,7.54870382904371,171.485485069079));
#45531=CARTESIAN_POINT('',(-73.9667318408259,6.31261103702609,171.485485069079));
#45532=CARTESIAN_POINT('',(-73.9319567695917,6.14627830862634,171.485485069079));
#45533=CARTESIAN_POINT('',(-64.4948557181401,2.4488872837273,171.485485069079));
#45534=CARTESIAN_POINT('',(-76.6565310829785,7.40982146175055,171.485485069079));
#45535=CARTESIAN_POINT('',(-64.6577925771904,-15.1217749800782,171.485485069079));
#45536=CARTESIAN_POINT('',(-64.4948557181401,2.4488872837273,171.485485069079));
#45537=CARTESIAN_POINT('',(-83.3698713720824,-60.9942295498001,171.485485069079));
#45538=CARTESIAN_POINT('Origin',(-76.1376696617351,8.68180450729347,180.485485069079));
#45539=CARTESIAN_POINT('',(-75.2878441530478,10.7651423591035,177.485485069079));
#45540=CARTESIAN_POINT('',(-75.2878441530478,10.7651423591035,174.485485069079));
#45541=CARTESIAN_POINT('',(-75.2878441530478,10.7651423591035,180.985485069079));
#45542=CARTESIAN_POINT('',(-78.1205958486722,3.82068285307013,174.485485069079));
#45543=CARTESIAN_POINT('',(-76.1376696617351,8.68180450729347,174.485485069079));
#45544=CARTESIAN_POINT('',(-78.1205958486722,3.82068285307013,177.485485069079));
#45545=CARTESIAN_POINT('',(-78.1205958486722,3.82068285307013,180.485485069079));
#45546=CARTESIAN_POINT('',(-76.1376696617351,8.68180450729347,177.485485069079));
#45547=CARTESIAN_POINT('Origin',(-178.096445811705,1.62308776542128,180.485485069079));
#45548=CARTESIAN_POINT('',(-88.4637952304757,-42.7163749036655,174.485485069079));
#45549=CARTESIAN_POINT('Origin',(-178.096445811705,1.62308776542128,174.485485069079));
#45550=CARTESIAN_POINT('',(-88.4637952304757,-42.7163749036655,177.485485069079));
#45551=CARTESIAN_POINT('',(-88.4637952304757,-42.7163749036655,180.485485069079));
#45552=CARTESIAN_POINT('Origin',(-178.096445811705,1.62308776542128,177.485485069079));
#45553=CARTESIAN_POINT('Origin',(-88.4637952304757,-42.7163749036655,180.485485069079));
#45554=CARTESIAN_POINT('',(-113.298872866457,-103.599293529631,174.485485069079));
#45555=CARTESIAN_POINT('',(-88.4637952304757,-42.7163749036655,177.485485069079));
#45556=CARTESIAN_POINT('Origin',(-64.3046088901795,-18.2273525712768,180.485485069079));
#45557=CARTESIAN_POINT('',(-64.3046088901795,-18.2273525712768,178.985485069079));
#45558=CARTESIAN_POINT('',(-64.3046088901795,-18.2273525712768,178.785485069079));
#45559=CARTESIAN_POINT('',(-64.3046088901795,-18.2273525712768,180.485485069079));
#45560=CARTESIAN_POINT('',(-64.3046088901795,-18.2273525712768,178.985485069079));
#45561=CARTESIAN_POINT('',(-73.5957040846178,-41.004369859499,178.785485069079));
#45562=CARTESIAN_POINT('Origin',(-64.100606517944,3.77170156821119,180.485485069079));
#45563=CARTESIAN_POINT('',(-64.0976157548621,4.09421722445422,179.285485069079));
#45564=CARTESIAN_POINT('',(-64.067029466095,7.39255839147599,179.285485069079));
#45565=CARTESIAN_POINT('',(-64.100606517944,3.77170156821119,179.285485069079));
#45566=CARTESIAN_POINT('',(-64.067029466095,7.39255839147599,179.485485069079));
#45567=CARTESIAN_POINT('',(-64.067029466095,7.39255839147599,180.485485069079));
#45568=CARTESIAN_POINT('',(-64.3024536808101,-17.9949407268459,179.485485069079));
#45569=CARTESIAN_POINT('',(-64.100606517944,3.77170156821119,179.485485069079));
#45570=CARTESIAN_POINT('Origin',(-64.2669244479286,-14.1635660759491,178.985485069037));
#45571=CARTESIAN_POINT('',(-64.1113219987316,2.61617362315227,178.785485069079));
#45572=CARTESIAN_POINT('',(-64.1303313887531,0.566253342026285,178.785485069079));
#45573=CARTESIAN_POINT('',(-64.0969218480186,4.16904622791266,179.310798599544));
#45574=CARTESIAN_POINT('Origin',(-76.1376696617351,8.68180450729347,170.985485069079));
#45575=CARTESIAN_POINT('',(-73.0571341974619,7.42520677607053,170.985485069079));
#45576=CARTESIAN_POINT('',(-65.5950181087078,4.38129500943137,170.985485069079));
#45577=CARTESIAN_POINT('',(-76.1376696617351,8.68180450729347,170.985485069079));
#45578=CARTESIAN_POINT('Origin',(-65.6361368403207,-0.0528357944954805,
172.485485069087));
#45579=CARTESIAN_POINT('Origin',(-72.0398282687001,2.55932829637862,172.485485069078));
#45580=CARTESIAN_POINT('Origin',(-69.9391102914966,14.1820463536532,180.985485069079));
#45581=CARTESIAN_POINT('',(-73.0571341974619,7.42520677607053,180.985485069079));
#45582=CARTESIAN_POINT('',(-65.5950181087078,4.38129500943137,180.985485069079));
#45583=CARTESIAN_POINT('',(-76.1376696617351,8.68180450729347,180.985485069079));
#45584=CARTESIAN_POINT('',(-65.5045147937286,14.14092331283,180.985485069079));
#45585=CARTESIAN_POINT('',(-65.5045147937286,14.14092331283,180.985485069079));
#45586=CARTESIAN_POINT('',(-74.2800401190792,13.2744910851909,180.985485069079));
#45587=CARTESIAN_POINT('Origin',(-69.9391102914966,14.1820463536532,180.985485069079));
#45588=CARTESIAN_POINT('',(-73.2641860378138,8.41555694081837,180.985485069079));
#45589=CARTESIAN_POINT('Origin',(-69.9391102914966,14.1820463536532,170.985485069079));
#45590=CARTESIAN_POINT('',(-74.2800401190792,13.2744910851909,170.985485069079));
#45591=CARTESIAN_POINT('',(-65.5045147937286,14.14092331283,170.985485069079));
#45592=CARTESIAN_POINT('Origin',(-69.9391102914966,14.1820463536532,170.985485069079));
#45593=CARTESIAN_POINT('',(-65.5045147937286,14.14092331283,170.985485069079));
#45594=CARTESIAN_POINT('',(-74.2800401190792,13.2744910851909,170.985485069079));
#45595=CARTESIAN_POINT('Origin',(-76.1376696617351,8.68180450729347,180.985485069079));
#45596=CARTESIAN_POINT('Origin',(-65.6361368403178,-0.0528357944828661,
179.485485069077));
#45597=CARTESIAN_POINT('Origin',(-72.0398282686983,2.55932829637348,179.485485069079));
#45598=CARTESIAN_POINT('Origin',(-75.7482946184945,12.9675241082264,180.985485069079));
#45599=CARTESIAN_POINT('',(-75.0082722890301,9.42792149152613,179.485485069079));
#45600=CARTESIAN_POINT('',(-75.5631600798882,12.0820066431433,179.485485069079));
#45601=CARTESIAN_POINT('',(-75.7482946184945,12.9675241082264,179.485485069079));
#45602=CARTESIAN_POINT('',(-75.5631600798882,12.0820066431433,172.485485069079));
#45603=CARTESIAN_POINT('',(-75.5631600798882,12.0820066431433,180.985485069079));
#45604=CARTESIAN_POINT('',(-75.0082722890301,9.42792149152613,172.485485069079));
#45605=CARTESIAN_POINT('',(-75.7482946184945,12.9675241082264,172.485485069079));
#45606=CARTESIAN_POINT('Origin',(-74.1899511896153,5.51380783648853,174.485485069067));
#45607=CARTESIAN_POINT('Origin',(-74.1899511896128,5.51380783647723,177.485485069089));
#45608=CARTESIAN_POINT('Origin',(-178.096445811705,1.62308776542128,178.785485069079));
#45609=CARTESIAN_POINT('Origin',(-107.523469003812,-101.851499334574,178.785485069079));
#45610=CARTESIAN_POINT('',(-86.9127681729002,-43.414973163782,178.785485069079));
#45611=CARTESIAN_POINT('',(-84.1699457474323,-36.6909742706479,178.785485069079));
#45612=CARTESIAN_POINT('',(-76.4138381126899,3.50385663167992,178.785485069079));
#45613=CARTESIAN_POINT('Origin',(-178.096445811705,1.62308776542128,178.785485069079));
#45614=CARTESIAN_POINT('',(-74.9692357361314,7.04528340827526,178.785485069079));
#45615=CARTESIAN_POINT('',(-91.5773692205345,-33.6693724619818,178.785485069079));
#45616=CARTESIAN_POINT('',(-76.5433132241656,7.68737379261679,178.785485069079));
#45617=CARTESIAN_POINT('Origin',(-178.096445811705,1.62308776542128,173.185485069079));
#45618=CARTESIAN_POINT('Origin',(-107.523469003812,-101.851499334574,173.185485069079));
#45619=CARTESIAN_POINT('',(-74.9692357361314,7.04528340827526,173.185485069079));
#45620=CARTESIAN_POINT('',(-76.5433132241656,7.68737379261679,173.185485069079));
#45621=CARTESIAN_POINT('',(-76.4138381126899,3.50385663167992,173.185485069079));
#45622=CARTESIAN_POINT('',(-91.5773692205345,-33.6693724619818,173.185485069079));
#45623=CARTESIAN_POINT('',(-86.9127681729002,-43.414973163782,173.185485069079));
#45624=CARTESIAN_POINT('Origin',(-178.096445811705,1.62308776542128,173.185485069079));
#45625=CARTESIAN_POINT('',(-84.1699457474323,-36.6909742706479,173.185485069079));
#45626=CARTESIAN_POINT('Origin',(-74.5635921737009,8.03971412295194,180.485485069079));
#45627=CARTESIAN_POINT('',(-74.4503743148881,8.31726645381818,172.685485069079));
#45628=CARTESIAN_POINT('',(-74.3439843284204,8.57808033101511,172.582962524415));
#45629=CARTESIAN_POINT('',(-73.5174599342508,10.6042957578474,172.685485069079));
#45630=CARTESIAN_POINT('',(-74.5635921737009,8.03971412295194,172.685485069079));
#45631=CARTESIAN_POINT('',(-73.5174599342508,10.6042957578474,179.285485069079));
#45632=CARTESIAN_POINT('',(-73.5174599342508,10.6042957578474,180.985485069079));
#45633=CARTESIAN_POINT('',(-74.4503743148881,8.31726645381818,179.285485069079));
#45634=CARTESIAN_POINT('',(-74.5635921737009,8.03971412295194,179.285485069079));
#45635=CARTESIAN_POINT('',(-74.3439843284204,8.57808033101511,179.388007613743));
#45636=CARTESIAN_POINT('',(-76.4138381126899,3.50385663167992,178.785485069079));
#45637=CARTESIAN_POINT('Origin',(-178.096445811705,1.62308776542128,180.485485069079));
#45638=CARTESIAN_POINT('',(-86.9127681729002,-43.414973163782,178.785485069079));
#45639=CARTESIAN_POINT('Origin',(-86.8897177424414,-43.358465288007,180.485485069079));
#45640=CARTESIAN_POINT('Origin',(-75.9180618164546,9.22017071535663,172.582962524415));
#45641=CARTESIAN_POINT('',(-76.0244518029223,8.95935683815971,172.685485069079));
#45642=CARTESIAN_POINT('Origin',(-69.9391102914966,14.1820463536532,179.285485069079));
#45643=CARTESIAN_POINT('',(-73.6644795614854,11.3075056969888,179.285485069079));
#45644=CARTESIAN_POINT('',(-74.0842728524905,13.3154200154528,179.285485069079));
#45645=CARTESIAN_POINT('',(-71.4758555404412,10.4147323427326,179.285485069079));
#45646=CARTESIAN_POINT('',(-76.0244518029223,8.95935683815971,179.285485069079));
#45647=CARTESIAN_POINT('Origin',(-69.9391102914966,14.1820463536532,172.685485069079));
#45648=CARTESIAN_POINT('',(-73.6644795614854,11.3075056969888,172.685485069079));
#45649=CARTESIAN_POINT('',(-71.4758555404412,10.4147323427326,172.685485069079));
#45650=CARTESIAN_POINT('',(-74.0842728524905,13.3154200154528,172.685485069079));
#45651=CARTESIAN_POINT('Origin',(-75.9180618164546,9.22017071535663,179.388007613743));
#45652=CARTESIAN_POINT('Origin',(-74.0842728524905,13.3154200154528,180.985485069079));
#45653=CARTESIAN_POINT('',(-73.6644795614854,11.3075056969888,180.985485069079));
#45654=CARTESIAN_POINT('Origin',(-178.096445811705,1.62308776542128,174.485485069079));
#45655=CARTESIAN_POINT('Ctrl Pts',(-85.7265587833611,-43.9488769757557,
171.485485069079));
#45656=CARTESIAN_POINT('Ctrl Pts',(-85.803250652307,-43.914368625268,171.485485069079));
#45657=CARTESIAN_POINT('Ctrl Pts',(-85.8800425344643,-43.8798139862072,
171.489021188661));
#45658=CARTESIAN_POINT('Ctrl Pts',(-85.9565889693217,-43.8453679850229,
171.496095119029));
#45659=CARTESIAN_POINT('Ctrl Pts',(-86.033153479375,-43.8109138499754,171.503170719791));
#45660=CARTESIAN_POINT('Ctrl Pts',(-86.1094719448409,-43.7765686004695,
171.513785775505));
#45661=CARTESIAN_POINT('Ctrl Pts',(-86.1852015595645,-43.7424860901274,
171.527889918968));
#45662=CARTESIAN_POINT('Ctrl Pts',(-86.2609375075804,-43.708400729454,171.541995241965));
#45663=CARTESIAN_POINT('Ctrl Pts',(-86.3360840355133,-43.674578343957,171.559590124626));
#45664=CARTESIAN_POINT('Ctrl Pts',(-86.4103083068289,-43.6411687240148,
171.580573167936));
#45665=CARTESIAN_POINT('Ctrl Pts',(-86.484621793816,-43.6077189465657,171.601581432327));
#45666=CARTESIAN_POINT('Ctrl Pts',(-86.5580103545068,-43.5746831116226,
171.625985823891));
#45667=CARTESIAN_POINT('Ctrl Pts',(-86.6301569692901,-43.5422046082181,
171.653635642269));
#45668=CARTESIAN_POINT('Ctrl Pts',(-86.6794632456137,-43.5200082228679,
171.672532018619));
#45669=CARTESIAN_POINT('Ctrl Pts',(-86.7281898183943,-43.498071998044,171.692943178902));
#45670=CARTESIAN_POINT('Ctrl Pts',(-86.7762416508316,-43.4764391924131,
171.714808688551));
#45671=CARTESIAN_POINT('Ctrl Pts',(-86.844202757917,-43.4458432849216,171.745733716116));
#45672=CARTESIAN_POINT('Ctrl Pts',(-86.9112560532974,-43.4156547293774,
171.779771728895));
#45673=CARTESIAN_POINT('Ctrl Pts',(-86.9770837908681,-43.3860162755525,
171.816822321779));
#45674=CARTESIAN_POINT('Ctrl Pts',(-87.0428464088205,-43.3564071413559,
171.85383626263));
#45675=CARTESIAN_POINT('Ctrl Pts',(-87.1073854308492,-43.3273472093682,
171.89385665786));
#45676=CARTESIAN_POINT('Ctrl Pts',(-87.1703999907691,-43.2989723048369,
171.936734325967));
#45677=CARTESIAN_POINT('Ctrl Pts',(-87.1969931361074,-43.2869976443596,
171.954829383065));
#45678=CARTESIAN_POINT('Ctrl Pts',(-87.2233150134355,-43.2751448897427,
171.973432729157));
#45679=CARTESIAN_POINT('Ctrl Pts',(-87.2493441620514,-43.263423779529,171.992530657435));
#45680=CARTESIAN_POINT('Ctrl Pts',(-87.3074800086726,-43.2372447955113,
172.035185691818));
#45681=CARTESIAN_POINT('Ctrl Pts',(-87.3638206194771,-43.2118725332094,
172.080056350151));
#45682=CARTESIAN_POINT('Ctrl Pts',(-87.4184018693449,-43.1872918753659,
172.127088854887));
#45683=CARTESIAN_POINT('Ctrl Pts',(-87.4733030268523,-43.162567147164,172.174397023108));
#45684=CARTESIAN_POINT('Ctrl Pts',(-87.5264247429931,-43.1386430837505,
172.223892902332));
#45685=CARTESIAN_POINT('Ctrl Pts',(-87.5777782826842,-43.1155145981015,
172.275566687581));
#45686=CARTESIAN_POINT('Ctrl Pts',(-87.6066127988569,-43.1025281769607,
172.304581018539));
#45687=CARTESIAN_POINT('Ctrl Pts',(-87.6348893538779,-43.0897927850127,
172.334282751313));
#45688=CARTESIAN_POINT('Ctrl Pts',(-87.6626054251485,-43.0773093641887,
172.364675456255));
#45689=CARTESIAN_POINT('Ctrl Pts',(-87.7022875141167,-43.0594364048168,
172.408189777231));
#45690=CARTESIAN_POINT('Ctrl Pts',(-87.7409436157031,-43.0420261537913,
172.453262073559));
#45691=CARTESIAN_POINT('Ctrl Pts',(-87.7783597289956,-43.0251734587016,
172.4997017108));
#45692=CARTESIAN_POINT('Ctrl Pts',(-87.815731883462,-43.0083405632284,172.546086787806));
#45693=CARTESIAN_POINT('Ctrl Pts',(-87.8518666337329,-42.9920640480807,
172.593835653644));
#45694=CARTESIAN_POINT('Ctrl Pts',(-87.8865850093306,-42.9764244448045,
172.642721841606));
#45695=CARTESIAN_POINT('Ctrl Pts',(-87.9213372796397,-42.9607695729615,
172.691655755973));
#45696=CARTESIAN_POINT('Ctrl Pts',(-87.9546701380456,-42.9457529674742,
172.741728816459));
#45697=CARTESIAN_POINT('Ctrl Pts',(-87.9864429746324,-42.9314395340925,
172.792682837345));
#45698=CARTESIAN_POINT('Ctrl Pts',(-87.9921769878195,-42.9288564025695,
172.80187846037));
#45699=CARTESIAN_POINT('Ctrl Pts',(-87.9978603003912,-42.9262961287167,
172.811102703421));
#45700=CARTESIAN_POINT('Ctrl Pts',(-88.0034922301876,-42.9237590351675,
172.820353957677));
#45701=CARTESIAN_POINT('Ctrl Pts',(-88.0423527552536,-42.9062529953147,
172.88418795613));
#45702=CARTESIAN_POINT('Ctrl Pts',(-88.0788588190602,-42.8898062504737,
172.949452352716));
#45703=CARTESIAN_POINT('Ctrl Pts',(-88.1130345979563,-42.8744094619404,
173.016132724375));
#45704=CARTESIAN_POINT('Ctrl Pts',(-88.1471669345133,-42.8590322449437,
173.082728335673));
#45705=CARTESIAN_POINT('Ctrl Pts',(-88.1789752565884,-42.8447021739146,
173.150737019641));
#45706=CARTESIAN_POINT('Ctrl Pts',(-88.2084421665376,-42.8314268668266,
173.220170227426));
#45707=CARTESIAN_POINT('Ctrl Pts',(-88.2248095428287,-42.8240531059923,
173.258736858297));
#45708=CARTESIAN_POINT('Ctrl Pts',(-88.2404537681471,-42.8170050788906,
173.29774338966));
#45709=CARTESIAN_POINT('Ctrl Pts',(-88.2553657482793,-42.8102865845098,
173.337194006733));
#45710=CARTESIAN_POINT('Ctrl Pts',(-88.2785508339243,-42.7998406969589,
173.398531664609));
#45711=CARTESIAN_POINT('Ctrl Pts',(-88.2999340259369,-42.7902077310875,
173.460870943718));
#45712=CARTESIAN_POINT('Ctrl Pts',(-88.3194011434631,-42.7814372835972,
173.523931455552));
#45713=CARTESIAN_POINT('Ctrl Pts',(-88.3388862024838,-42.7726587529926,
173.587050085894));
#45714=CARTESIAN_POINT('Ctrl Pts',(-88.3564514902963,-42.7647443979481,
173.650890795394));
#45715=CARTESIAN_POINT('Ctrl Pts',(-88.3720283006514,-42.7577252737347,
173.715155412108));
#45716=CARTESIAN_POINT('Ctrl Pts',(-88.386961771976,-42.7509960469049,173.776765830993));
#45717=CARTESIAN_POINT('Ctrl Pts',(-88.4000678620873,-42.7450895338618,
173.838765365943));
#45718=CARTESIAN_POINT('Ctrl Pts',(-88.4113270034268,-42.7400163854414,
173.900882979141));
#45719=CARTESIAN_POINT('Ctrl Pts',(-88.4248392494687,-42.7339280322006,
173.975431157173));
#45720=CARTESIAN_POINT('Ctrl Pts',(-88.4357556434908,-42.7290082994433,
174.050459862041));
#45721=CARTESIAN_POINT('Ctrl Pts',(-88.4440715753402,-42.7252609302257,
174.125976729112));
#45722=CARTESIAN_POINT('Ctrl Pts',(-88.4523200024512,-42.7215439803506,
174.200880586548));
#45723=CARTESIAN_POINT('Ctrl Pts',(-88.4580100367288,-42.7189804288886,
174.276265478641));
#45724=CARTESIAN_POINT('Ctrl Pts',(-88.4610900430369,-42.7175931561194,
174.352140154751));
#45725=CARTESIAN_POINT('Ctrl Pts',(-88.4628875726858,-42.7167835266303,
174.396421551042));
#45726=CARTESIAN_POINT('Ctrl Pts',(-88.4637952304757,-42.7163749036655,
174.440869736792));
#45727=CARTESIAN_POINT('Ctrl Pts',(-88.4637952304757,-42.7163749036655,
174.485485069079));
#45728=CARTESIAN_POINT('Ctrl Pts',(-75.1094485830761,3.25967012829815,171.485485069079));
#45729=CARTESIAN_POINT('Ctrl Pts',(-75.1120445846317,3.2601578535513,171.485485069079));
#45730=CARTESIAN_POINT('Ctrl Pts',(-75.1146405871344,3.26064556863604,171.485488417755));
#45731=CARTESIAN_POINT('Ctrl Pts',(-75.5167168146379,3.33618265944911,171.486525721311));
#45732=CARTESIAN_POINT('Ctrl Pts',(-75.9126646258982,3.41031403917456,171.566843725105));
#45733=CARTESIAN_POINT('Ctrl Pts',(-76.6469980011459,3.54738856602921,171.876254905816));
#45734=CARTESIAN_POINT('Ctrl Pts',(-76.9795047377048,3.60924302566342,172.10107561908));
#45735=CARTESIAN_POINT('Ctrl Pts',(-77.5328013082622,3.71195743403252,172.66315582424));
#45736=CARTESIAN_POINT('Ctrl Pts',(-77.7505284531588,3.75226045795544,172.992534367449));
#45737=CARTESIAN_POINT('Ctrl Pts',(-78.0441240514199,3.80656466012662,173.711715425967));
#45738=CARTESIAN_POINT('Ctrl Pts',(-78.1196409565064,3.82050645968902,174.092743833336));
#45739=CARTESIAN_POINT('Ctrl Pts',(-78.1205928503534,3.82068229920291,174.480597840799));
#45740=CARTESIAN_POINT('Ctrl Pts',(-78.1205958486722,3.82068285307013,174.483041537554));
#45741=CARTESIAN_POINT('Ctrl Pts',(-78.1205958486722,3.82068285307013,174.485485069079));
#45742=CARTESIAN_POINT('Origin',(-73.3598858593218,7.54870382904371,174.485485069079));
#45743=CARTESIAN_POINT('Ctrl Pts',(-75.0082722890301,9.42792149152613,172.485485069079));
#45744=CARTESIAN_POINT('Ctrl Pts',(-74.9739694602182,9.26384754701334,172.380688709692));
#45745=CARTESIAN_POINT('Ctrl Pts',(-74.9285618899177,9.10219402976686,172.281030806539));
#45746=CARTESIAN_POINT('Ctrl Pts',(-74.7471063051629,8.54399815677015,171.960847918504));
#45747=CARTESIAN_POINT('Ctrl Pts',(-74.5448580111294,8.09335437334894,171.758213612547));
#45748=CARTESIAN_POINT('Ctrl Pts',(-74.1813523460724,7.1343272986673,171.523884315342));
#45749=CARTESIAN_POINT('Ctrl Pts',(-74.0316751243507,6.62324141552802,171.485485069079));
#45750=CARTESIAN_POINT('Ctrl Pts',(-73.9319567695917,6.14627830862634,171.485485069079));
#45751=CARTESIAN_POINT('Origin',(-178.096445811705,1.62308776542128,177.485485069079));
#45752=CARTESIAN_POINT('Ctrl Pts',(-88.4637952304757,-42.7163749036655,
177.485485069079));
#45753=CARTESIAN_POINT('Ctrl Pts',(-88.4637952304757,-42.7163749036655,
177.561790921156));
#45754=CARTESIAN_POINT('Ctrl Pts',(-88.4611428086215,-42.7175691207664,
177.63760722595));
#45755=CARTESIAN_POINT('Ctrl Pts',(-88.4559170665894,-42.7199234808925,
177.712938143183));
#45756=CARTESIAN_POINT('Ctrl Pts',(-88.4506407020019,-42.7223006480621,
177.788998802434));
#45757=CARTESIAN_POINT('Ctrl Pts',(-88.4427409408535,-42.725860535365,177.86456540467));
#45758=CARTESIAN_POINT('Ctrl Pts',(-88.4322503736512,-42.7305879883129,
177.939647769675));
#45759=CARTESIAN_POINT('Ctrl Pts',(-88.4261504565341,-42.7333368455101,
177.983305676312));
#45760=CARTESIAN_POINT('Ctrl Pts',(-88.4191736653467,-42.7364808333816,
178.026799902097));
#45761=CARTESIAN_POINT('Ctrl Pts',(-88.4113189409649,-42.7400200182287,
178.070131638527));
#45762=CARTESIAN_POINT('Ctrl Pts',(-88.3995732954023,-42.7453123758946,
178.134928211008));
#45763=CARTESIAN_POINT('Ctrl Pts',(-88.3858176127608,-42.751511672146,178.199596284079));
#45764=CARTESIAN_POINT('Ctrl Pts',(-88.3700751037746,-42.7586054082518,
178.263828290739));
#45765=CARTESIAN_POINT('Ctrl Pts',(-88.3543457755428,-42.7656932049744,
178.32800651777));
#45766=CARTESIAN_POINT('Ctrl Pts',(-88.3366330233926,-42.7736739130754,
178.391748902742));
#45767=CARTESIAN_POINT('Ctrl Pts',(-88.3170073313624,-42.7825157579229,
178.45475847167));
#45768=CARTESIAN_POINT('Ctrl Pts',(-88.2981763416785,-42.7909995703079,
178.515216596696));
#45769=CARTESIAN_POINT('Ctrl Pts',(-88.2775846114719,-42.8002760222853,
178.574999737149));
#45770=CARTESIAN_POINT('Ctrl Pts',(-88.255333885622,-42.8103009400199,178.633860422541));
#45771=CARTESIAN_POINT('Ctrl Pts',(-88.2285124211434,-42.8223851738887,
178.704812255441));
#45772=CARTESIAN_POINT('Ctrl Pts',(-88.1993250780218,-42.8355342384889,
178.774328445248));
#45773=CARTESIAN_POINT('Ctrl Pts',(-88.1678143700804,-42.8497302730071,
178.842430176088));
#45774=CARTESIAN_POINT('Ctrl Pts',(-88.1362149276743,-42.8639662836987,
178.910723682074));
#45775=CARTESIAN_POINT('Ctrl Pts',(-88.1022787041779,-42.8792552966842,
178.977595470867));
#45776=CARTESIAN_POINT('Ctrl Pts',(-88.0660039857381,-42.8955974879037,
179.043046798095));
#45777=CARTESIAN_POINT('Ctrl Pts',(-88.045866981765,-42.9046694472095,179.079380467745));
#45778=CARTESIAN_POINT('Ctrl Pts',(-88.0250085722305,-42.9140662704144,
179.115275982884));
#45779=CARTESIAN_POINT('Ctrl Pts',(-88.0034231363848,-42.9237901608107,
179.150729671394));
#45780=CARTESIAN_POINT('Ctrl Pts',(-87.9722169216766,-42.937848056777,179.201985315421));
#45781=CARTESIAN_POINT('Ctrl Pts',(-87.9394301197629,-42.9526188574974,
179.252409455835));
#45782=CARTESIAN_POINT('Ctrl Pts',(-87.9051958767024,-42.9680407049136,
179.301739114946));
#45783=CARTESIAN_POINT('Ctrl Pts',(-87.870989601021,-42.9834499535803,179.351028474603));
#45784=CARTESIAN_POINT('Ctrl Pts',(-87.8353385026604,-42.9995090818352,
179.399224732454));
#45785=CARTESIAN_POINT('Ctrl Pts',(-87.7984148583883,-43.016140288081,179.446095415752));
#45786=CARTESIAN_POINT('Ctrl Pts',(-87.7614367362052,-43.0327960323536,
179.493035253029));
#45787=CARTESIAN_POINT('Ctrl Pts',(-87.7231826255935,-43.0500254153442,
179.538645243775));
#45788=CARTESIAN_POINT('Ctrl Pts',(-87.6838608886981,-43.0677358823089,
179.582727629355));
#45789=CARTESIAN_POINT('Ctrl Pts',(-87.6767708756422,-43.0709292163761,
179.590676024161));
#45790=CARTESIAN_POINT('Ctrl Pts',(-87.6696462380143,-43.0741381562752,
179.598574856602));
#45791=CARTESIAN_POINT('Ctrl Pts',(-87.6624883060175,-43.077362115076,179.606423103847));
#45792=CARTESIAN_POINT('Ctrl Pts',(-87.6131318343259,-43.0995924507871,
179.660539543226));
#45793=CARTESIAN_POINT('Ctrl Pts',(-87.5620001392908,-43.1226209376601,
179.712467127506));
#45794=CARTESIAN_POINT('Ctrl Pts',(-87.5090998705986,-43.1464453560287,
179.762217973346));
#45795=CARTESIAN_POINT('Ctrl Pts',(-87.4564279354805,-43.1701669409953,
179.811754079474));
#45796=CARTESIAN_POINT('Ctrl Pts',(-87.4020020892567,-43.1946778346095,
179.859132678972));
#45797=CARTESIAN_POINT('Ctrl Pts',(-87.3457992427768,-43.2199879417789,
179.904325581094));
#45798=CARTESIAN_POINT('Ctrl Pts',(-87.3141559279581,-43.2342380330006,
179.929770079353));
#45799=CARTESIAN_POINT('Ctrl Pts',(-87.2819488300374,-43.2487416676317,
179.954520963863));
#45800=CARTESIAN_POINT('Ctrl Pts',(-87.2491707291509,-43.2635018775903,
179.978566720226));
#45801=CARTESIAN_POINT('Ctrl Pts',(-87.1874231391168,-43.2913072527857,
180.023864265409));
#45802=CARTESIAN_POINT('Ctrl Pts',(-87.1240278699442,-43.3198535458025,
180.066374884163));
#45803=CARTESIAN_POINT('Ctrl Pts',(-87.0592774397836,-43.3490083205518,
180.10592960246));
#45804=CARTESIAN_POINT('Ctrl Pts',(-86.994455720103,-43.3781951943912,180.145527870073));
#45805=CARTESIAN_POINT('Ctrl Pts',(-86.9282763051401,-43.4079917064379,
180.182163520666));
#45806=CARTESIAN_POINT('Ctrl Pts',(-86.8610515278968,-43.4382572944597,
180.215715122154));
#45807=CARTESIAN_POINT('Ctrl Pts',(-86.8328807003895,-43.450940217253,180.229775062802));
#45808=CARTESIAN_POINT('Ctrl Pts',(-86.8045264883465,-43.463705436197,180.243294021659));
#45809=CARTESIAN_POINT('Ctrl Pts',(-86.7760125604202,-43.4765423282938,
180.256265681589));
#45810=CARTESIAN_POINT('Ctrl Pts',(-86.6840444637611,-43.517946113006,180.298104143037));
#45811=CARTESIAN_POINT('Ctrl Pts',(-86.5897272059914,-43.5604047951258,
180.334559206954));
#45812=CARTESIAN_POINT('Ctrl Pts',(-86.4935381712521,-43.6037025304365,
180.365327483151));
#45813=CARTESIAN_POINT('Ctrl Pts',(-86.4176500184837,-43.6378621949002,
180.389602055099));
#45814=CARTESIAN_POINT('Ctrl Pts',(-86.3405974644073,-43.6725438472567,
180.410337515834));
#45815=CARTESIAN_POINT('Ctrl Pts',(-86.2626305571894,-43.7076351215567,
180.427400457632));
#45816=CARTESIAN_POINT('Ctrl Pts',(-86.2032719335862,-43.7343511965846,
180.44039100421));
#45817=CARTESIAN_POINT('Ctrl Pts',(-86.1434246486064,-43.7612859572302,
180.451240234448));
#45818=CARTESIAN_POINT('Ctrl Pts',(-86.0833635482303,-43.7883156486128,
180.459893197225));
#45819=CARTESIAN_POINT('Ctrl Pts',(-86.0231931259934,-43.8153945388302,
180.46856190993));
#45820=CARTESIAN_POINT('Ctrl Pts',(-85.9628085830272,-43.8425685124351,
180.475026292058));
#45821=CARTESIAN_POINT('Ctrl Pts',(-85.9024912617655,-43.8697111008618,
180.479283238523));
#45822=CARTESIAN_POINT('Ctrl Pts',(-85.8436965864612,-43.8961685038115,
180.48343272295));
#45823=CARTESIAN_POINT('Ctrl Pts',(-85.7849662058798,-43.9225959131722,
180.485485069079));
#45824=CARTESIAN_POINT('Ctrl Pts',(-85.7265587833611,-43.9488769757557,
180.485485069079));
#45825=CARTESIAN_POINT('Ctrl Pts',(-78.1205958486722,3.82068285307014,177.485485069079));
#45826=CARTESIAN_POINT('Ctrl Pts',(-78.1205958486722,3.82068285307014,177.487928596335));
#45827=CARTESIAN_POINT('Ctrl Pts',(-78.1205928503639,3.82068229920484,177.490372288819));
#45828=CARTESIAN_POINT('Ctrl Pts',(-78.1196409581911,3.82050646000022,177.878226291952));
#45829=CARTESIAN_POINT('Ctrl Pts',(-78.044124054763,3.80656466074426,178.259254699594));
#45830=CARTESIAN_POINT('Ctrl Pts',(-77.7505284596663,3.75226045915992,178.978435759267));
#45831=CARTESIAN_POINT('Ctrl Pts',(-77.532801316253,3.71195743551325,179.307814303359));
#45832=CARTESIAN_POINT('Ctrl Pts',(-76.9795047482519,3.60924302762411,179.86989451086));
#45833=CARTESIAN_POINT('Ctrl Pts',(-76.6469980127308,3.54738856818747,180.094715225556));
#45834=CARTESIAN_POINT('Ctrl Pts',(-75.9126646351845,3.41031404091361,180.404126411066));
#45835=CARTESIAN_POINT('Ctrl Pts',(-75.5167168218597,3.33618265904544,180.484444416827));
#45836=CARTESIAN_POINT('Ctrl Pts',(-75.1146405870959,3.2606455686755,180.485481720403));
#45837=CARTESIAN_POINT('Ctrl Pts',(-75.1120445846825,3.26015785356084,180.485485069079));
#45838=CARTESIAN_POINT('Ctrl Pts',(-75.1094485830761,3.25967012829816,180.485485069079));
#45839=CARTESIAN_POINT('Origin',(-90.3736629061554,-34.16038275589,177.485485069079));
#45840=CARTESIAN_POINT('Ctrl Pts',(-73.9319567695917,6.14627830862636,180.485485069079));
#45841=CARTESIAN_POINT('Ctrl Pts',(-74.0316751243507,6.62324141552803,180.485485069079));
#45842=CARTESIAN_POINT('Ctrl Pts',(-74.1813523460724,7.1343272986673,180.447085822817));
#45843=CARTESIAN_POINT('Ctrl Pts',(-74.5448580111294,8.09335437334895,180.212756525611));
#45844=CARTESIAN_POINT('Ctrl Pts',(-74.7471063051629,8.54399815677015,180.010122219654));
#45845=CARTESIAN_POINT('Ctrl Pts',(-74.9285618899177,9.10219402976687,179.68993933162));
#45846=CARTESIAN_POINT('Ctrl Pts',(-74.9739694602182,9.26384754701335,179.590281428466));
#45847=CARTESIAN_POINT('Ctrl Pts',(-75.0082722890301,9.42792149152614,179.485485069079));
#45848=CARTESIAN_POINT('Origin',(-85.6860114280623,-43.8494755819152,174.485485069079));
#45849=CARTESIAN_POINT('Origin',(-82.9662394330532,-37.1819845645561,177.485485069079));
#45850=CARTESIAN_POINT('Origin',(-74.2800401190792,13.2744910851909,172.485485069079));
#45851=CARTESIAN_POINT('',(-75.7482946184945,12.9675241082264,172.485485069079));
#45852=CARTESIAN_POINT('',(-75.7482946184945,12.9675241082264,172.485485069079));
#45853=CARTESIAN_POINT('Origin',(-74.2800401190792,13.2744910851909,172.485485069079));
#45854=CARTESIAN_POINT('Origin',(-65.6935007913861,-17.6608022321519,172.985485069079));
#45855=CARTESIAN_POINT('Ctrl Pts',(-64.30245368081,-17.9949407268459,172.485485069079));
#45856=CARTESIAN_POINT('Ctrl Pts',(-64.3021058587946,-17.95743255836,172.446326101961));
#45857=CARTESIAN_POINT('Ctrl Pts',(-64.3033770800788,-17.9191055129556,
172.407568629705));
#45858=CARTESIAN_POINT('Ctrl Pts',(-64.3167498663848,-17.7106704190456,
172.203844459849));
#45859=CARTESIAN_POINT('Ctrl Pts',(-64.3568840214925,-17.5200526030795,
172.048524450343));
#45860=CARTESIAN_POINT('Ctrl Pts',(-64.4530685529843,-17.0982909105767,
171.800345132073));
#45861=CARTESIAN_POINT('Ctrl Pts',(-64.5071684893368,-16.8667300414478,
171.707442565609));
#45862=CARTESIAN_POINT('Ctrl Pts',(-64.6326468132148,-16.1395439177394,
171.512810422578));
#45863=CARTESIAN_POINT('Ctrl Pts',(-64.6622884122446,-15.6065934538952,
171.485485069079));
#45864=CARTESIAN_POINT('Ctrl Pts',(-64.6577925771903,-15.1217749800779,
171.485485069079));
#45865=CARTESIAN_POINT('Origin',(-69.9391102914966,14.1820463536532,172.485485069079));
#45866=CARTESIAN_POINT('',(-64.0045792842181,14.1270140601776,172.485485069079));
#45867=CARTESIAN_POINT('Origin',(-69.9391102914966,14.1820463536532,172.485485069079));
#45868=CARTESIAN_POINT('Origin',(-65.5045147937286,14.14092331283,172.485485069079));
#45869=CARTESIAN_POINT('Origin',(-65.6005420274545,3.78561082086359,172.485485069079));
#45870=CARTESIAN_POINT('',(-64.100606517944,3.77170156821119,172.485485069079));
#45871=CARTESIAN_POINT('Origin',(-74.2800401190792,13.2744910851909,179.485485069079));
#45872=CARTESIAN_POINT('',(-75.7482946184945,12.9675241082264,179.485485069079));
#45873=CARTESIAN_POINT('Origin',(-74.2800401190792,13.2744910851909,179.485485069079));
#45874=CARTESIAN_POINT('',(-75.7482946184945,12.9675241082265,179.485485069079));
#45875=CARTESIAN_POINT('Origin',(-74.9845959858244,-40.4378195203742,178.985485069079));
#45876=CARTESIAN_POINT('Ctrl Pts',(-64.6577925771903,-15.121774980078,180.485485069079));
#45877=CARTESIAN_POINT('Ctrl Pts',(-64.6622884122446,-15.6065934538952,
180.485485069079));
#45878=CARTESIAN_POINT('Ctrl Pts',(-64.6326468132148,-16.1395439177395,
180.45815971558));
#45879=CARTESIAN_POINT('Ctrl Pts',(-64.5071684893368,-16.8667300414478,
180.26352757255));
#45880=CARTESIAN_POINT('Ctrl Pts',(-64.4530685529843,-17.0982909105767,
180.170625006086));
#45881=CARTESIAN_POINT('Ctrl Pts',(-64.3568840214925,-17.5200526030795,
179.922445687816));
#45882=CARTESIAN_POINT('Ctrl Pts',(-64.3167498663848,-17.7106704190457,
179.767125678309));
#45883=CARTESIAN_POINT('Ctrl Pts',(-64.3033770800788,-17.9191055129557,
179.563401508453));
#45884=CARTESIAN_POINT('Ctrl Pts',(-64.3021058587946,-17.95743255836,179.524644036198));
#45885=CARTESIAN_POINT('Ctrl Pts',(-64.30245368081,-17.9949407268459,179.485485069079));
#45886=CARTESIAN_POINT('Origin',(-69.9391102914966,14.1820463536532,179.485485069079));
#45887=CARTESIAN_POINT('',(-64.0045792842181,14.1270140601776,179.485485069079));
#45888=CARTESIAN_POINT('Origin',(-65.5045147937286,14.14092331283,179.485485069079));
#45889=CARTESIAN_POINT('Origin',(-69.9391102914966,14.1820463536532,179.485485069079));
#45890=CARTESIAN_POINT('Origin',(-65.5045147937286,14.14092331283,179.485485069079));
#45891=CARTESIAN_POINT('',(-64.100606517944,3.77170156821119,179.485485069079));
#45892=CARTESIAN_POINT('Origin',(-107.523469003812,-101.851499334574,361.145530749938));
#45893=CARTESIAN_POINT('Origin',(-76.9710398341703,12.6563024191807,172.485485069079));
#45894=CARTESIAN_POINT('',(-76.9710398341703,12.6563024191807,179.485485069079));
#45895=CARTESIAN_POINT('',(-76.9710398341703,12.6563024191807,172.485485069079));
#45896=CARTESIAN_POINT('Origin',(-73.1927245087776,21.9188007238304,172.485485069079));
#45897=CARTESIAN_POINT('Origin',(-73.1927245087776,21.9188007238304,179.485485069079));
#47698=UNCERTAINTY_MEASURE_WITH_UNIT(LENGTH_MEASURE(0.01),#47718,
'DISTANCE_ACCURACY_VALUE',
'Maximum model space distance between geometric entities at asserted c
onnectivities');
#47703=UNCERTAINTY_MEASURE_WITH_UNIT(LENGTH_MEASURE(0.01),#47718,
'DISTANCE_ACCURACY_VALUE',
'Maximum model space distance between geometric entities at asserted c
onnectivities');
#47712=(
GEOMETRIC_REPRESENTATION_CONTEXT(3)
GLOBAL_UNCERTAINTY_ASSIGNED_CONTEXT((#47698))
GLOBAL_UNIT_ASSIGNED_CONTEXT((#47718,#47720,#47721))
REPRESENTATION_CONTEXT('','3D')
);
#47717=(
GEOMETRIC_REPRESENTATION_CONTEXT(3)
GLOBAL_UNCERTAINTY_ASSIGNED_CONTEXT((#47703))
GLOBAL_UNIT_ASSIGNED_CONTEXT((#47718,#47720,#47721))
REPRESENTATION_CONTEXT('','3D')
);
#47718=(
LENGTH_UNIT()
NAMED_UNIT(*)
SI_UNIT(.MILLI.,.METRE.)
);
#47720=(
NAMED_UNIT(*)
PLANE_ANGLE_UNIT()
SI_UNIT($,.RADIAN.)
);
#47721=(
NAMED_UNIT(*)
SI_UNIT($,.STERADIAN.)
SOLID_ANGLE_UNIT()
);
#47730=SHAPE_DEFINITION_REPRESENTATION(#47743,#47768);
#47743=PRODUCT_DEFINITION_SHAPE('',$,#47782);
#47768=SHAPE_REPRESENTATION('',(#9703),#47712);
#47773=PRODUCT_DEFINITION_CONTEXT('part definition',#47814,'design');
#47782=PRODUCT_DEFINITION('Lower Handle','Lower Handle',#47795,#47773);
#47795=PRODUCT_DEFINITION_FORMATION('',$,#47824);
#47814=APPLICATION_CONTEXT(
'Core Data for Automotive Mechanical Design Process');
#47815=PRODUCT_CONTEXT('part definition',#47814,'mechanical');
#47824=PRODUCT('Lower Handle','Lower Handle',$,(#47815));
#47830=PRESENTATION_STYLE_ASSIGNMENT((#47832));
#47832=SURFACE_STYLE_USAGE(.BOTH.,#47834);
#47834=SURFACE_SIDE_STYLE('',(#47836));
#47836=SURFACE_STYLE_FILL_AREA(#47838);
#47838=FILL_AREA_STYLE('Opaque(202,209,238)',(#47840));
#47840=FILL_AREA_STYLE_COLOUR('Opaque(202,209,238)',#47842);
#47842=COLOUR_RGB('Opaque(202,209,238)', 0.66274510, 0.83137255, 0.94901961);
ENDSEC;
END-ISO-10303-21;
